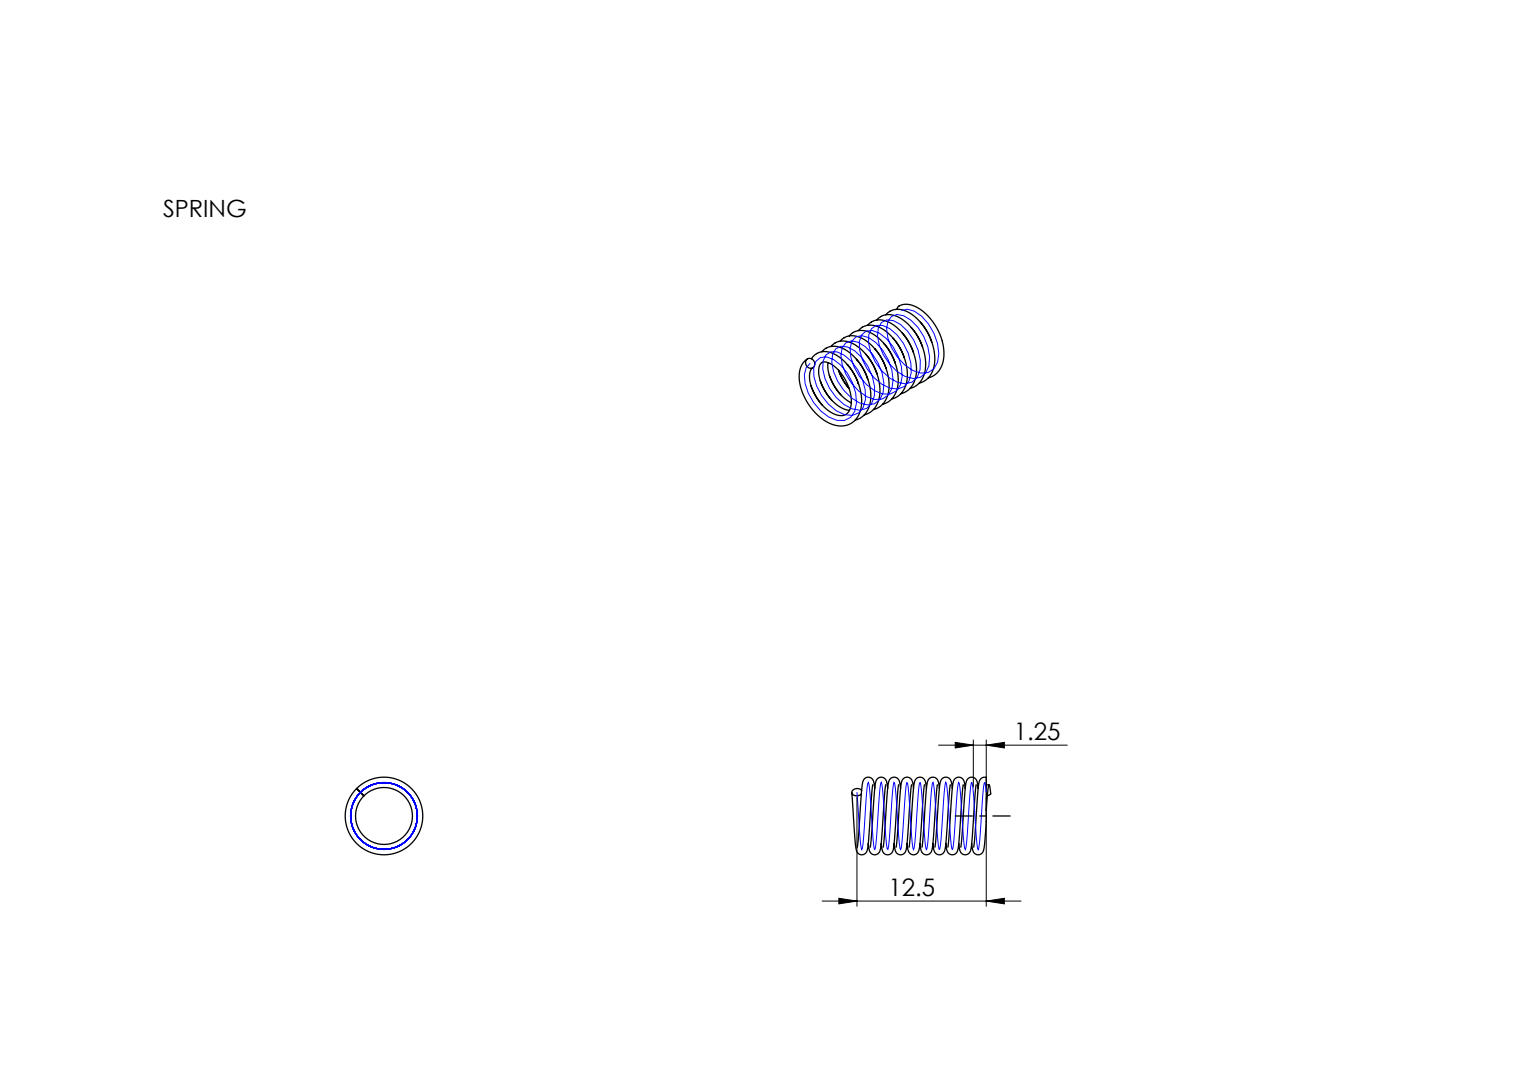
ISO-10303-21;
HEADER;
FILE_DESCRIPTION (('STEP AP214'),
    '1' );
FILE_NAME ('spring.step',
    '2026-10-05T05:16:24',
    ( '' ),
    ( '' ),
    'SwSTEP 2.0',
    'SolidWorks 2026',
    '' );
FILE_SCHEMA (( 'AUTOMOTIVE_DESIGN' ));
ENDSEC;

DATA;
#9=MANIFOLD_SOLID_BREP ( 'Cavity1', #19917 ) ;
#49=CARTESIAN_POINT ( 'NONE',  ( 1.553300858899129944, -11.24999999999998934, 14.70312500000000355 ) ) ;
#65=CARTESIAN_POINT ( 'NONE',  ( 1.200186371490529202, -4.775308065498752974, 18.23624329374151642 ) ) ;
#121=CARTESIAN_POINT ( 'NONE',  ( 2.651650429449539104, -4.848349570550432475, 24.31250000000000000 ) ) ;
#168=CARTESIAN_POINT ( 'NONE',  ( -2.749999999999998224, -7.500000000000015987, 20.09375000000000000 ) ) ;
#179=CARTESIAN_POINT ( 'NONE',  ( 2.750000000000001776, -7.499999999999984013, 18.21875000000000000 ) ) ;
#188=CARTESIAN_POINT ( 'NONE',  ( -2.651650429449565305, -4.848349570550461785, 26.50000000000000355 ) ) ;
#239=CARTESIAN_POINT ( 'NONE',  ( -2.651650429449535551, -10.15165042944956753, 18.68750000000000000 ) ) ;
#270=CARTESIAN_POINT ( 'NONE',  ( -1.987747218494660295, -5.598659921968651254, 17.49813170625848713 ) ) ;
#281=CARTESIAN_POINT ( 'NONE',  ( 1.200186371490561621, -10.22469193450123193, 19.45125670625849068 ) ) ;
#289=CARTESIAN_POINT ( 'NONE',  ( 1.492201783934598236, -11.27530806549875031, 21.20499329374151998 ) ) ;
#294=CARTESIAN_POINT ( 'NONE',  ( 2.608446859217924629, -10.19485399968118422, 24.87686829374151642 ) ) ;
#339=CARTESIAN_POINT ( 'NONE',  ( 1.653273178848927064E-15, -7.500000000000000000, 0.000000000000000000 ) ) ;
#384=CARTESIAN_POINT ( 'NONE',  ( -1.614399933863656544, -3.775308065498769405, 16.32625670625849068 ) ) ;
#392=CARTESIAN_POINT ( 'NONE',  ( -2.608446859217889546, -10.19485399968121264, 18.43563170625848713 ) ) ;
#407=CARTESIAN_POINT ( 'NONE',  ( -2.724691934501246582, -6.299813628509474128, 20.42374329374152353 ) ) ;
#454=CIRCLE ( 'NONE', #72316, 0.4999999999999994449 ) ;
#493=CARTESIAN_POINT ( 'NONE',  ( 1.553300858899087311, -3.749999999999992006, 14.23437500000000355 ) ) ;
#511=CARTESIAN_POINT ( 'NONE',  ( 1.901340078031373171, -9.487747218494639867, 23.62686829374151287 ) ) ;
#518=PRESENTATION_STYLE_ASSIGNMENT (( #82052 ) ) ;
#612=LINE ( 'NONE', #14123, #34562 ) ;
#615=CARTESIAN_POINT ( 'NONE',  ( 1.139087296526029469, -10.24999999999999467, 19.70312500000000355 ) ) ;
#678=CARTESIAN_POINT ( 'NONE',  ( -3.749999999999997335, -7.500000000000021316, 22.59375000000000355 ) ) ;
#710=CARTESIAN_POINT ( 'NONE',  ( -1.901340078031346525, -9.487747218494661183, 19.68563170625849068 ) ) ;
#722=CARTESIAN_POINT ( 'NONE',  ( 1.987747218494664292, -9.401340078031346081, 19.37313170625848713 ) ) ;
#729=CARTESIAN_POINT ( 'NONE',  ( -0.06109907496450878162, -11.25000000000000000, 23.78311829374151998 ) ) ;
#735=CARTESIAN_POINT ( 'NONE',  ( 2.694853999681185108, -4.891553140782077591, 23.31436829374150932 ) ) ;
#817=CARTESIAN_POINT ( 'NONE',  ( -3.749999999999996447, -7.561099074964554134, 17.34188170625849068 ) ) ;
#828=CARTESIAN_POINT ( 'NONE',  ( 0.06109907496455496689, -11.24999999999999822, 15.77938170625848890 ) ) ;
#843=CARTESIAN_POINT ( 'NONE',  ( -2.749999999999999112, -7.438900925035484057, 22.84561829374151642 ) ) ;
#933=CARTESIAN_POINT ( 'NONE',  ( -2.651650429449565305, -4.848349570550461785, 14.00000000000000000 ) ) ;
#939=ORIENTED_EDGE ( 'NONE', *, *, #22476, .F. ) ;
#948=CARTESIAN_POINT ( 'NONE',  ( 1.492201783934598236, -11.27530806549875031, 14.95499329374151642 ) ) ;
#956=CARTESIAN_POINT ( 'NONE',  ( 1.799775606325937360E-14, -10.25000000000000000, 14.78125000000000178 ) ) ;
#1056=CARTESIAN_POINT ( 'NONE',  ( 2.749999999999995115, -6.360912703473971419, 21.89062500000000355 ) ) ;
#1072=CARTESIAN_POINT ( 'NONE',  ( 3.749999999999992006, -5.946699141100872943, 24.39062500000000000 ) ) ;
#1084=ORIENTED_EDGE ( 'NONE', *, *, #14407, .T. ) ;
#1153=CARTESIAN_POINT ( 'NONE',  ( -0.06109907496454585613, -4.750000000000000000, 23.90438170625849068 ) ) ;
#1163=CARTESIAN_POINT ( 'NONE',  ( -1.077988221561460236, -10.27530806549876452, 19.60750670625849068 ) ) ;
#1170=CARTESIAN_POINT ( 'NONE',  ( -2.694853999681181556, -10.10844685921792241, 22.68936829374151287 ) ) ;
#1174=CARTESIAN_POINT ( 'NONE',  ( 3.724691934501251023, -9.114399933863618131, 23.54874329374151642 ) ) ;
#1253=CARTESIAN_POINT ( 'NONE',  ( -1.929879867024197893E-14, -3.750000000000000000, 25.40625000000000000 ) ) ;
#1262=CARTESIAN_POINT ( 'NONE',  ( 3.775308065498768517, -8.992201783934554271, 15.54500670625849246 ) ) ;
#1279=CARTESIAN_POINT ( 'NONE',  ( 2.724691934501250135, -8.700186371490531201, 22.29874329374151642 ) ) ;
#1388=CARTESIAN_POINT ( 'NONE',  ( 1.200186371490529202, -4.775308065498752974, 23.23624329374151642 ) ) ;
#1504=CARTESIAN_POINT ( 'NONE',  ( -2.749999999999991562, -8.639087296526025028, 26.26562500000000000 ) ) ;
#1601=CARTESIAN_POINT ( 'NONE',  ( 2.775308065498768517, -8.577988221561467341, 20.54500670625849068 ) ) ;
#1612=CARTESIAN_POINT ( 'NONE',  ( -0.06109907496454585613, -4.750000000000000000, 25.15438170625849068 ) ) ;
#1621=CARTESIAN_POINT ( 'NONE',  ( -1.553300858899125059, -3.750000000000009326, 15.32812500000000355 ) ) ;
#1630=CARTESIAN_POINT ( 'NONE',  ( -2.651650429449535551, -10.15165042944956753, 17.43750000000000000 ) ) ;
#1705=CARTESIAN_POINT ( 'NONE',  ( 0.06109907496455496689, -11.24999999999999822, 22.02938170625849068 ) ) ;
#1714=CARTESIAN_POINT ( 'NONE',  ( 1.614399933863660985, -11.22469193450123193, 20.70125670625849423 ) ) ;
#1729=CARTESIAN_POINT ( 'NONE',  ( 1.200186371490529202, -4.775308065498752974, 21.98624329374151642 ) ) ;
#1738=ADVANCED_FACE ( 'NONE', ( #45379 ), #86854, .F. ) ;
#1805=CARTESIAN_POINT ( 'NONE',  ( -3.749999999999997335, -7.500000000000021316, 15.09375000000000000 ) ) ;
#1815=CARTESIAN_POINT ( 'NONE',  ( 2.651650429449569302, -10.15165042944953733, 14.62500000000000000 ) ) ;
#1830=CARTESIAN_POINT ( 'NONE',  ( -1.492201783934593573, -3.724691934501250135, 13.07999329374151642 ) ) ;
#1834=CARTESIAN_POINT ( 'NONE',  ( 2.749999999999995115, -6.360912703473971419, 18.14062500000000711 ) ) ;
#1842=CARTESIAN_POINT ( 'NONE',  ( 2.749999999999995115, -6.360912703473971419, 14.39062500000000000 ) ) ;
#1941=CARTESIAN_POINT ( 'NONE',  ( -2.749999999999998224, -7.500000000000015987, 23.84375000000000000 ) ) ;
#2009=CARTESIAN_POINT ( 'NONE',  ( -1.553300858899125059, -3.750000000000009326, 25.32812500000000355 ) ) ;
#2036=CARTESIAN_POINT ( 'NONE',  ( -1.200186371490556958, -4.775308065498765409, 21.32625670625849423 ) ) ;
#2039=CARTESIAN_POINT ( 'NONE',  ( 3.155571303690441365, -7.975156536449540035, 14.00000000000001066 ) ) ;
#2049=CARTESIAN_POINT ( 'NONE',  ( -1.077988221561460236, -10.27530806549876452, 22.10750670625849068 ) ) ;
#2058=CARTESIAN_POINT ( 'NONE',  ( 1.553300858899087311, -3.749999999999992006, 15.48437500000000178 ) ) ;
#2063=CARTESIAN_POINT ( 'NONE',  ( -3.749999999999997335, -7.500000000000021316, 15.09375000000000000 ) ) ;
#2098=CARTESIAN_POINT ( 'NONE',  ( -1.553300858899081538, -11.25000000000000711, 19.85937500000000355 ) ) ;
#2139=CARTESIAN_POINT ( 'NONE',  ( 3.749999999999999556, -7.438900925035446754, 19.21688170625848358 ) ) ;
#2151=CARTESIAN_POINT ( 'NONE',  ( -2.608446859217889546, -10.19485399968121264, 23.43563170625848713 ) ) ;
#2163=CARTESIAN_POINT ( 'NONE',  ( 1.492201783934598236, -11.27530806549875031, 13.70499329374151287 ) ) ;
#2236=CARTESIAN_POINT ( 'NONE',  ( 2.320192649118979489E-14, -11.25000000000000000, 16.03125000000000000 ) ) ;
#2245=CARTESIAN_POINT ( 'NONE',  ( -2.651650429449565305, -4.848349570550461785, 16.50000000000000000 ) ) ;
#2259=CARTESIAN_POINT ( 'NONE',  ( -0.06109907496450878162, -11.25000000000000000, 15.03311829374151287 ) ) ;
#2263=CARTESIAN_POINT ( 'NONE',  ( -2.749999999999991562, -8.639087296526025028, 23.76562499999999645 ) ) ;
#2267=CARTESIAN_POINT ( 'NONE',  ( -1.139087296525992388, -10.25000000000000711, 16.10937500000000355 ) ) ;
#2366=CARTESIAN_POINT ( 'NONE',  ( -2.749999999999998224, -7.500000000000015987, 25.09374999999999645 ) ) ;
#2438=CARTESIAN_POINT ( 'NONE',  ( -3.750000000000007550, -5.946699141100917352, 25.17187500000000000 ) ) ;
#2469=CARTESIAN_POINT ( 'NONE',  ( 2.750000000000001332, -7.438900925035452083, 24.21688170625849068 ) ) ;
#2481=CARTESIAN_POINT ( 'NONE',  ( 1.901340078031349856, -5.512252781505337929, 22.81063170625848713 ) ) ;
#2490=CARTESIAN_POINT ( 'NONE',  ( 2.320192649118979489E-14, -11.25000000000000000, 17.28125000000000000 ) ) ;
#2495=CARTESIAN_POINT ( 'NONE',  ( 1.553300858899129944, -11.24999999999998934, 15.95312500000000000 ) ) ;
#2531=CARTESIAN_POINT ( 'NONE',  ( -3.749999999999988454, -9.053300858899127945, 20.01562500000000355 ) ) ;
#2572=CARTESIAN_POINT ( 'NONE',  ( -2.694853999681210865, -4.891553140782108677, 22.49813170625848713 ) ) ;
#2582=CARTESIAN_POINT ( 'NONE',  ( 1.492201783934554493, -3.724691934501233703, 22.73250670625849068 ) ) ;
#2598=CARTESIAN_POINT ( 'NONE',  ( -2.694853999681181556, -10.10844685921792241, 15.18936829374151465 ) ) ;
#2674=CARTESIAN_POINT ( 'NONE',  ( 2.651650429449569302, -10.15165042944953733, 15.87500000000000000 ) ) ;
#2686=CARTESIAN_POINT ( 'NONE',  ( 2.651650429449539104, -4.848349570550432475, 16.81250000000000000 ) ) ;
#2699=CARTESIAN_POINT ( 'NONE',  ( 3.775308065498752086, -6.007798216065404873, 19.64249329374151642 ) ) ;
#2703=CARTESIAN_POINT ( 'NONE',  ( 1.799775606325937360E-14, -10.25000000000000000, 24.78125000000000000 ) ) ;
#2806=CARTESIAN_POINT ( 'NONE',  ( -1.901340078031369618, -5.512252781505359245, 13.00186829374151465 ) ) ;
#2874=CARTESIAN_POINT ( 'NONE',  ( -1.553300858899081760, -11.25000000000000888, 23.60937500000000711 ) ) ;
#2909=CARTESIAN_POINT ( 'NONE',  ( 2.775308065498768517, -8.577988221561467341, 21.79500670625849068 ) ) ;
#2922=CARTESIAN_POINT ( 'NONE',  ( -2.724691934501232371, -8.700186371490559623, 23.51375670625848713 ) ) ;
#2933=CARTESIAN_POINT ( 'NONE',  ( -1.929879867024197893E-14, -3.750000000000000000, 16.65625000000000000 ) ) ;
#2939=CARTESIAN_POINT ( 'NONE',  ( 1.553300858899129944, -11.24999999999998934, 17.20312500000000000 ) ) ;
#2978=CARTESIAN_POINT ( 'NONE',  ( -1.553300858899081538, -11.25000000000000711, 23.60937500000000711 ) ) ;
#3018=CARTESIAN_POINT ( 'NONE',  ( -3.724691934501229262, -9.114399933863657211, 18.51375670625849068 ) ) ;
#3026=CARTESIAN_POINT ( 'NONE',  ( -3.749999999999996447, -7.561099074964554134, 22.34188170625849068 ) ) ;
#3042=CARTESIAN_POINT ( 'NONE',  ( 1.987747218494642309, -5.598659921968629050, 24.56436829374151287 ) ) ;
#3124=CARTESIAN_POINT ( 'NONE',  ( -3.749999999999997335, -7.500000000000021316, 18.84375000000000000 ) ) ;
#3133=CARTESIAN_POINT ( 'NONE',  ( 3.749999999999992006, -5.946699141100872943, 18.14062500000000711 ) ) ;
#3148=CARTESIAN_POINT ( 'NONE',  ( 2.608446859217924629, -10.19485399968118422, 16.12686829374151287 ) ) ;
#3153=CARTESIAN_POINT ( 'NONE',  ( 1.139087296525997273, -4.749999999999992895, 22.98437500000000000 ) ) ;
#3158=CARTESIAN_POINT ( 'NONE',  ( -1.944543648263014957, -5.555456351737005249, 19.00000000000000000 ) ) ;
#3258=CARTESIAN_POINT ( 'NONE',  ( -2.749999999999999112, -7.438900925035484057, 15.34561829374151465 ) ) ;
#3365=CARTESIAN_POINT ( 'NONE',  ( 2.750000000000008438, -8.639087296525996607, 14.54687500000000178 ) ) ;
#3375=CARTESIAN_POINT ( 'NONE',  ( 2.750000000000001332, -7.438900925035452083, 24.21688170625849068 ) ) ;
#3385=CARTESIAN_POINT ( 'NONE',  ( 1.553300858899129944, -11.24999999999998934, 14.70312500000000355 ) ) ;
#3389=CARTESIAN_POINT ( 'NONE',  ( -3.750000000000008438, -5.946699141100917352, 15.17187500000000000 ) ) ;
#3427=CARTESIAN_POINT ( 'NONE',  ( 2.651650429449539104, -4.848349570550432475, 20.56250000000000000 ) ) ;
#3433=CARTESIAN_POINT ( 'NONE',  ( 3.749999999999992006, -5.946699141100872943, 15.64062500000000178 ) ) ;
#3465=CARTESIAN_POINT ( 'NONE',  ( -2.608446859217889546, -10.19485399968121264, 20.93563170625849068 ) ) ;
#3474=CARTESIAN_POINT ( 'NONE',  ( 0.06109907496455496689, -11.24999999999999822, 22.02938170625849068 ) ) ;
#3487=CARTESIAN_POINT ( 'NONE',  ( 2.608446859217924629, -10.19485399968118422, 16.12686829374151287 ) ) ;
#3569=CARTESIAN_POINT ( 'NONE',  ( 3.749999999999992006, -5.946699141100872943, 14.39062500000000178 ) ) ;
#3579=CARTESIAN_POINT ( 'NONE',  ( 3.750000000000009770, -9.053300858899081760, 17.04687500000000000 ) ) ;
#3594=CARTESIAN_POINT ( 'NONE',  ( 0.06109907496451268821, -3.749999999999999556, 16.90811829374151287 ) ) ;
#3600=CARTESIAN_POINT ( 'NONE',  ( 1.799775606325937360E-14, -10.25000000000000000, 26.03125000000000000 ) ) ;
#3606=CARTESIAN_POINT ( 'NONE',  ( 1.944543648262996083, -5.555456351736983045, 19.31250000000000000 ) ) ;
#3697=CARTESIAN_POINT ( 'NONE',  ( -2.749999999999999112, -7.438900925035484057, 14.09561829374151642 ) ) ;
#3812=CARTESIAN_POINT ( 'NONE',  ( 1.139087296525997273, -4.749999999999992895, 15.48437500000000178 ) ) ;
#3822=CARTESIAN_POINT ( 'NONE',  ( 1.944543648263018731, -9.444543648262994751, 17.12500000000000000 ) ) ;
#3831=CARTESIAN_POINT ( 'NONE',  ( -1.553300858899081538, -11.25000000000000711, 19.85937500000000355 ) ) ;
#3867=CARTESIAN_POINT ( 'NONE',  ( -3.750000000000008438, -5.946699141100917352, 22.67187500000000355 ) ) ;
#3875=CARTESIAN_POINT ( 'NONE',  ( 1.553300858899086867, -3.749999999999992006, 16.73437500000000000 ) ) ;
#3889=CARTESIAN_POINT ( 'NONE',  ( 1.269044939587668397, -4.511073634464840332, 13.80223852175840626 ) ) ;
#3905=CARTESIAN_POINT ( 'NONE',  ( -2.608446859217889546, -10.19485399968121264, 23.43563170625848713 ) ) ;
#3915=CARTESIAN_POINT ( 'NONE',  ( -2.694853999681210865, -4.891553140782108677, 23.74813170625849068 ) ) ;
#3929=CARTESIAN_POINT ( 'NONE',  ( -2.749999999999999112, -7.438900925035484057, 25.34561829374151642 ) ) ;
#4008=CARTESIAN_POINT ( 'NONE',  ( 2.651650429449569302, -10.15165042944953733, 23.37500000000000000 ) ) ;
#4019=CARTESIAN_POINT ( 'NONE',  ( -3.749999999999997335, -7.500000000000021316, 17.59375000000000000 ) ) ;
#4037=CARTESIAN_POINT ( 'NONE',  ( 1.944543648262996083, -5.555456351736983045, 25.56250000000000355 ) ) ;
#4043=CARTESIAN_POINT ( 'NONE',  ( -2.749999999999998224, -7.500000000000015987, 18.84375000000000000 ) ) ;
#4141=CARTESIAN_POINT ( 'NONE',  ( -2.724691934501246582, -6.299813628509474128, 14.17374329374151287 ) ) ;
#4261=CARTESIAN_POINT ( 'NONE',  ( 2.749999999999995115, -6.360912703473971419, 15.64062500000000178 ) ) ;
#4269=CARTESIAN_POINT ( 'NONE',  ( 1.139087296526029469, -10.24999999999999467, 17.20312500000000000 ) ) ;
#4277=CARTESIAN_POINT ( 'NONE',  ( -3.749999999999988454, -9.053300858899127945, 21.26562500000000000 ) ) ;
#4328=CARTESIAN_POINT ( 'NONE',  ( -2.651650429449565305, -4.848349570550461785, 16.50000000000000000 ) ) ;
#4364=CARTESIAN_POINT ( 'NONE',  ( 3.775308065498768517, -8.992201783934554271, 23.04500670625849068 ) ) ;
#4374=CARTESIAN_POINT ( 'NONE',  ( -0.06109907496455085213, -3.750000000000000888, 23.90438170625849068 ) ) ;
#4387=CARTESIAN_POINT ( 'NONE',  ( 2.694853999681185108, -4.891553140782077591, 19.56436829374151287 ) ) ;
#4469=CARTESIAN_POINT ( 'NONE',  ( -3.749999999999997335, -7.500000000000021316, 20.09375000000000000 ) ) ;
#4482=CARTESIAN_POINT ( 'NONE',  ( 1.553300858899129944, -11.24999999999998934, 23.45312500000000000 ) ) ;
#4499=CARTESIAN_POINT ( 'NONE',  ( -2.775308065498752086, -8.577988221561495763, 17.76749329374151287 ) ) ;
#4504=CARTESIAN_POINT ( 'NONE',  ( 1.944543648263018731, -9.444543648262994751, 18.37500000000000355 ) ) ;
#4599=CARTESIAN_POINT ( 'NONE',  ( -2.775308065498752086, -8.577988221561495763, 17.76749329374151287 ) ) ;
#4715=CARTESIAN_POINT ( 'NONE',  ( -1.139087296526025916, -4.750000000000006217, 14.07812500000000178 ) ) ;
#4725=CARTESIAN_POINT ( 'NONE',  ( 1.987747218494664292, -9.401340078031346081, 26.87313170625849423 ) ) ;
#4733=CARTESIAN_POINT ( 'NONE',  ( -1.929879867024197893E-14, -3.750000000000000000, 21.65625000000000355 ) ) ;
#4783=CARTESIAN_POINT ( 'NONE',  ( -3.749999999999997335, -7.500000000000021316, 16.34375000000000000 ) ) ;
#4816=CARTESIAN_POINT ( 'NONE',  ( 2.608446859217893099, -4.805146000318787358, 26.56063170625849068 ) ) ;
#4826=CARTESIAN_POINT ( 'NONE',  ( -1.614399933863656544, -3.775308065498769405, 26.32625670625849068 ) ) ;
#4839=CARTESIAN_POINT ( 'NONE',  ( -3.724691934501248802, -5.885600066136383646, 17.92374329374151287 ) ) ;
#4926=CARTESIAN_POINT ( 'NONE',  ( 2.651650429449569302, -10.15165042944953733, 19.62500000000000000 ) ) ;
#4935=CARTESIAN_POINT ( 'NONE',  ( 2.320192649118979489E-14, -11.25000000000000000, 23.53125000000000000 ) ) ;
#4943=CARTESIAN_POINT ( 'NONE',  ( 2.952004793765244717, -6.965521097154411478, 14.00000000000000178 ) ) ;
#4951=CARTESIAN_POINT ( 'NONE',  ( 1.987747218494642309, -5.598659921968629050, 15.81436829374151465 ) ) ;
#4956=CARTESIAN_POINT ( 'NONE',  ( 1.944543648262996083, -5.555456351736983045, 16.81250000000000000 ) ) ;
#5043=CARTESIAN_POINT ( 'NONE',  ( 1.200186371490529202, -4.775308065498752974, 15.73624329374151998 ) ) ;
#5153=CARTESIAN_POINT ( 'NONE',  ( 2.750000000000001332, -7.438900925035452083, 25.46688170625849423 ) ) ;
#5162=CARTESIAN_POINT ( 'NONE',  ( 1.077988221561464899, -4.724691934501233703, 26.48250670625848713 ) ) ;
#5171=CARTESIAN_POINT ( 'NONE',  ( 3.750000000000009770, -9.053300858899081760, 22.04687500000000000 ) ) ;
#5214=CARTESIAN_POINT ( 'NONE',  ( 3.750000000000000888, -7.499999999999978684, 25.71875000000000000 ) ) ;
#5252=CARTESIAN_POINT ( 'NONE',  ( -1.987747218494660295, -5.598659921968651254, 14.99813170625848713 ) ) ;
#5265=CARTESIAN_POINT ( 'NONE',  ( 1.614399933863660985, -11.22469193450123193, 24.45125670625849423 ) ) ;
#5274=CARTESIAN_POINT ( 'NONE',  ( -1.614399933863613468, -11.22469193450124969, 20.11124329374151642 ) ) ;
#5280=CARTESIAN_POINT ( 'NONE',  ( 3.724691934501251023, -9.114399933863618131, 18.54874329374151642 ) ) ;
#5366=CARTESIAN_POINT ( 'NONE',  ( -1.929879867024197893E-14, -3.750000000000000000, 20.40625000000000000 ) ) ;
#5375=CARTESIAN_POINT ( 'NONE',  ( -3.749999999999988454, -9.053300858899127945, 25.01562500000000000 ) ) ;
#5395=CARTESIAN_POINT ( 'NONE',  ( 1.901340078031373171, -9.487747218494639867, 18.62686829374151642 ) ) ;
#5402=CARTESIAN_POINT ( 'NONE',  ( -1.139087296525992388, -10.25000000000000711, 24.85937500000000711 ) ) ;
#5500=CARTESIAN_POINT ( 'NONE',  ( 1.901340078031373171, -9.487747218494639867, 21.12686829374151287 ) ) ;
#5599=CARTESIAN_POINT ( 'NONE',  ( 2.749999999999995115, -6.360912703473971419, 19.39062500000000711 ) ) ;
#5608=CARTESIAN_POINT ( 'NONE',  ( -1.077988221561460236, -10.27530806549876452, 27.10750670625849423 ) ) ;
#5615=CARTESIAN_POINT ( 'NONE',  ( 2.320192649118979489E-14, -11.25000000000000000, 23.53125000000000000 ) ) ;
#5661=CARTESIAN_POINT ( 'NONE',  ( 3.750000000000009770, -9.053300858899081760, 19.54687500000000000 ) ) ;
#5691=CARTESIAN_POINT ( 'NONE',  ( 0.06109907496455496689, -11.24999999999999822, 23.27938170625849068 ) ) ;
#5707=CARTESIAN_POINT ( 'NONE',  ( -2.608446859217889546, -10.19485399968121264, 25.93563170625849423 ) ) ;
#5715=CARTESIAN_POINT ( 'NONE',  ( 2.608446859217924629, -10.19485399968118422, 17.37686829374151287 ) ) ;
#5721=CARTESIAN_POINT ( 'NONE',  ( 0.06109907496451268821, -3.749999999999999556, 18.15811829374151642 ) ) ;
#5808=CARTESIAN_POINT ( 'NONE',  ( -3.750000000000008438, -5.946699141100917352, 21.42187500000000000 ) ) ;
#5818=CARTESIAN_POINT ( 'NONE',  ( 3.749999999999992006, -5.946699141100872943, 23.14062500000000000 ) ) ;
#5833=CARTESIAN_POINT ( 'NONE',  ( -1.200186371490524317, -10.22469193450124791, 15.11124329374151287 ) ) ;
#5842=CARTESIAN_POINT ( 'NONE',  ( -1.139087296526025250, -4.750000000000006217, 22.82812500000000355 ) ) ;
#5942=CARTESIAN_POINT ( 'NONE',  ( -2.749999999999999112, -7.438900925035484057, 20.34561829374151287 ) ) ;
#6049=CARTESIAN_POINT ( 'NONE',  ( 1.944543648263018731, -9.444543648262994751, 20.87500000000000000 ) ) ;
#6057=CARTESIAN_POINT ( 'NONE',  ( 1.139087296525997273, -4.749999999999992895, 19.23437500000000355 ) ) ;
#6066=CARTESIAN_POINT ( 'NONE',  ( -1.553300858899125059, -3.750000000000009326, 24.07812500000000355 ) ) ;
#6114=CARTESIAN_POINT ( 'NONE',  ( 3.750000000000000888, -7.499999999999978684, 21.96875000000000355 ) ) ;
#6140=CARTESIAN_POINT ( 'NONE',  ( 1.200186371490561621, -10.22469193450123193, 16.95125670625848713 ) ) ;
#6154=CARTESIAN_POINT ( 'NONE',  ( -2.775308065498764964, -6.422011778438537988, 16.17000670625848713 ) ) ;
#6163=CARTESIAN_POINT ( 'NONE',  ( 3.775308065498752086, -6.007798216065404873, 23.39249329374151642 ) ) ;
#6168=CARTESIAN_POINT ( 'NONE',  ( -2.608446859217920633, -4.805146000318815780, 19.25186829374151287 ) ) ;
#6259=CARTESIAN_POINT ( 'NONE',  ( -3.749999999999996447, -7.561099074964554134, 16.09188170625848713 ) ) ;
#6267=CARTESIAN_POINT ( 'NONE',  ( -1.553300858899081538, -11.25000000000000711, 21.10937500000000711 ) ) ;
#6282=CARTESIAN_POINT ( 'NONE',  ( 0.06109907496451789238, -4.749999999999998224, 16.90811829374151287 ) ) ;
#6291=CARTESIAN_POINT ( 'NONE',  ( 1.799775606325937360E-14, -10.25000000000000000, 22.28125000000000355 ) ) ;
#6391=CARTESIAN_POINT ( 'NONE',  ( -0.06109907496451398579, -10.25000000000000178, 22.53311829374151642 ) ) ;
#6395=SURFACE_STYLE_FILL_AREA ( #48245 ) ;
#6490=CARTESIAN_POINT ( 'NONE',  ( -2.749999999999991562, -8.639087296526025028, 18.76562500000000000 ) ) ;
#6498=CARTESIAN_POINT ( 'NONE',  ( -1.409462824231155764E-14, -4.749999999999999112, 17.90625000000000000 ) ) ;
#6507=CARTESIAN_POINT ( 'NONE',  ( 2.651650429449539104, -4.848349570550432475, 24.31250000000000000 ) ) ;
#6556=CARTESIAN_POINT ( 'NONE',  ( -1.553300858899081760, -11.25000000000000888, 22.35937500000000355 ) ) ;
#6586=CARTESIAN_POINT ( 'NONE',  ( 0.06109907496454976272, -10.25000000000000000, 18.27938170625849068 ) ) ;
#6598=CARTESIAN_POINT ( 'NONE',  ( -1.901340078031346525, -9.487747218494661183, 17.18563170625848713 ) ) ;
#6604=CARTESIAN_POINT ( 'NONE',  ( -2.121320343559653487, -5.378679656440369605, 14.00000000000000178 ) ) ;
#6605=CARTESIAN_POINT ( 'NONE',  ( -2.608446859217920633, -4.805146000318815780, 24.25186829374150932 ) ) ;
#6610=CARTESIAN_POINT ( 'NONE',  ( -3.749999999999997780, -7.438900925035489387, 25.34561829374151642 ) ) ;
#6688=CARTESIAN_POINT ( 'NONE',  ( -1.553300858899081538, -11.25000000000000711, 24.85937500000001421 ) ) ;
#6696=CARTESIAN_POINT ( 'NONE',  ( 3.749999999999999556, -7.438900925035446754, 17.96688170625848713 ) ) ;
#6711=CARTESIAN_POINT ( 'NONE',  ( -2.724691934501246582, -6.299813628509474128, 21.67374329374151287 ) ) ;
#6719=CARTESIAN_POINT ( 'NONE',  ( 1.944543648262996083, -5.555456351736983045, 25.56250000000000355 ) ) ;
#6813=CARTESIAN_POINT ( 'NONE',  ( -2.749999999999999112, -7.438900925035484057, 22.84561829374151642 ) ) ;
#6871=CARTESIAN_POINT ( 'NONE',  ( 3.750000000000000888, -7.499999999999978684, 24.46875000000000000 ) ) ;
#6920=CARTESIAN_POINT ( 'NONE',  ( -2.749999999999991562, -8.639087296526025028, 17.51562500000000000 ) ) ;
#6931=CARTESIAN_POINT ( 'NONE',  ( -2.749999999999991562, -8.639087296526025028, 22.51562500000000000 ) ) ;
#6994=CARTESIAN_POINT ( 'NONE',  ( 1.553300858899129722, -11.24999999999999112, 18.45312499999999645 ) ) ;
#7021=CARTESIAN_POINT ( 'NONE',  ( -2.724691934501232371, -8.700186371490559623, 17.26375670625849068 ) ) ;
#7033=CARTESIAN_POINT ( 'NONE',  ( -1.200186371490556958, -4.775308065498765409, 18.82625670625848713 ) ) ;
#7042=CARTESIAN_POINT ( 'NONE',  ( 3.724691934501251023, -9.114399933863618131, 24.79874329374151998 ) ) ;
#7050=CARTESIAN_POINT ( 'NONE',  ( 3.775308065498752086, -6.007798216065404873, 23.39249329374151642 ) ) ;
#7137=CARTESIAN_POINT ( 'NONE',  ( 2.694853999681214862, -10.10844685921789043, 15.62313170625848890 ) ) ;
#7145=CARTESIAN_POINT ( 'NONE',  ( 3.775308065498768517, -8.992201783934554271, 16.79500670625849068 ) ) ;
#7162=CARTESIAN_POINT ( 'NONE',  ( -1.987747218494638313, -9.401340078031370950, 23.93936829374151642 ) ) ;
#7169=CARTESIAN_POINT ( 'NONE',  ( -2.749999999999991562, -8.639087296526026805, 22.51562500000000000 ) ) ;
#7252=CARTESIAN_POINT ( 'NONE',  ( 3.750000000000000888, -7.499999999999978684, 14.46875000000000000 ) ) ;
#7268=CARTESIAN_POINT ( 'NONE',  ( -1.901340078031369618, -5.512252781505359245, 19.25186829374151287 ) ) ;
#7326=CARTESIAN_POINT ( 'NONE',  ( 2.320192649118979489E-14, -11.25000000000000000, 24.78125000000000000 ) ) ;
#7378=CARTESIAN_POINT ( 'NONE',  ( -1.944543648262992530, -9.444543648263016067, 18.68750000000000000 ) ) ;
#7395=CARTESIAN_POINT ( 'NONE',  ( -1.553300858899125059, -3.750000000000009326, 25.32812500000000711 ) ) ;
#7445=CARTESIAN_POINT ( 'NONE',  ( 2.320192649118979489E-14, -11.25000000000000000, 21.03125000000000000 ) ) ;
#7477=CARTESIAN_POINT ( 'NONE',  ( -1.200186371490556958, -4.775308065498765409, 17.57625670625849068 ) ) ;
#7489=CARTESIAN_POINT ( 'NONE',  ( 1.077988221561464899, -4.724691934501233703, 16.48250670625849423 ) ) ;
#7497=CARTESIAN_POINT ( 'NONE',  ( -1.614399933863613468, -11.22469193450124969, 21.36124329374151642 ) ) ;
#7502=CARTESIAN_POINT ( 'NONE',  ( -2.694853999681181556, -10.10844685921792241, 22.68936829374151287 ) ) ;
#7568=AXIS2_PLACEMENT_3D ( 'NONE', #37517, #16371, #65873 ) ;
#7582=CARTESIAN_POINT ( 'NONE',  ( -3.724691934501229262, -9.114399933863657211, 17.26375670625849068 ) ) ;
#7591=CARTESIAN_POINT ( 'NONE',  ( 1.492201783934554493, -3.724691934501233703, 15.23250670625848713 ) ) ;
#7607=CARTESIAN_POINT ( 'NONE',  ( 1.987747218494642309, -5.598659921968629050, 20.81436829374151287 ) ) ;
#7614=CARTESIAN_POINT ( 'NONE',  ( -1.944543648263015179, -5.555456351737005249, 26.50000000000000355 ) ) ;
#7701=CARTESIAN_POINT ( 'NONE',  ( -2.651650429449565305, -4.848349570550461785, 15.25000000000000000 ) ) ;
#7718=CARTESIAN_POINT ( 'NONE',  ( 2.608446859217924629, -10.19485399968118422, 14.87686829374151465 ) ) ;
#7725=CARTESIAN_POINT ( 'NONE',  ( -1.139087296525992388, -10.25000000000000711, 14.85937500000000355 ) ) ;
#7816=CARTESIAN_POINT ( 'NONE',  ( 1.944543648263018731, -9.444543648262994751, 23.37500000000000000 ) ) ;
#7832=CARTESIAN_POINT ( 'NONE',  ( 2.651650429449569302, -10.15165042944953733, 25.87500000000000355 ) ) ;
#7915=CARTESIAN_POINT ( 'NONE',  ( -2.749999999999997780, -7.561099074964547917, 18.59188170625849068 ) ) ;
#7927=CARTESIAN_POINT ( 'NONE',  ( -1.901340078031346525, -9.487747218494661183, 18.43563170625848713 ) ) ;
#7934=CARTESIAN_POINT ( 'NONE',  ( 2.608446859217924629, -10.19485399968118422, 23.62686829374151287 ) ) ;
#7940=CARTESIAN_POINT ( 'NONE',  ( -3.749999999999997780, -7.438900925035489387, 21.59561829374151287 ) ) ;
#8024=CARTESIAN_POINT ( 'NONE',  ( 2.320192649118979489E-14, -11.25000000000000000, 26.03125000000000000 ) ) ;
#8033=CARTESIAN_POINT ( 'NONE',  ( -1.929879867024197893E-14, -3.750000000000000000, 25.40625000000000000 ) ) ;
#8050=CARTESIAN_POINT ( 'NONE',  ( 0.06109907496451789238, -4.749999999999998224, 20.65811829374151287 ) ) ;
#8155=CARTESIAN_POINT ( 'NONE',  ( -1.614399933863613468, -11.22469193450124969, 13.86124329374151820 ) ) ;
#8265=CARTESIAN_POINT ( 'NONE',  ( -1.139087296526025916, -4.750000000000006217, 24.07812500000000355 ) ) ;
#8362=CARTESIAN_POINT ( 'NONE',  ( 2.724691934501235036, -6.299813628509441266, 24.13875670625849068 ) ) ;
#8364=CARTESIAN_POINT ( 'NONE',  ( -1.790671178605550695, -4.201618623452029411, 14.00000000000000711 ) ) ;
#8373=CARTESIAN_POINT ( 'NONE',  ( -1.200186371490556958, -4.775308065498765409, 25.07625670625849423 ) ) ;
#8381=CARTESIAN_POINT ( 'NONE',  ( 2.320192649118979489E-14, -11.25000000000000000, 14.78125000000000178 ) ) ;
#8386=CARTESIAN_POINT ( 'NONE',  ( 3.775308065498752086, -6.007798216065404873, 22.14249329374151998 ) ) ;
#8470=CARTESIAN_POINT ( 'NONE',  ( 3.775308065498768517, -8.992201783934554271, 21.79500670625849068 ) ) ;
#8479=CARTESIAN_POINT ( 'NONE',  ( -3.724691934501229262, -9.114399933863657211, 17.26375670625849068 ) ) ;
#8494=CARTESIAN_POINT ( 'NONE',  ( -1.200186371490524317, -10.22469193450124791, 22.61124329374151287 ) ) ;
#8599=CARTESIAN_POINT ( 'NONE',  ( -1.077988221561493543, -4.724691934501247914, 23.07999329374151998 ) ) ;
#8605=CARTESIAN_POINT ( 'NONE',  ( -2.750000000000007105, -6.360912703474006946, 21.42187500000000000 ) ) ;
#8708=CARTESIAN_POINT ( 'NONE',  ( 1.799775606325937360E-14, -10.25000000000000000, 24.78125000000000000 ) ) ;
#8775=CARTESIAN_POINT ( 'NONE',  ( -2.651650429449565305, -4.848349570550461785, 25.25000000000000000 ) ) ;
#8807=CARTESIAN_POINT ( 'NONE',  ( 1.200186371490561621, -10.22469193450123193, 20.70125670625849423 ) ) ;
#8809=CARTESIAN_POINT ( 'NONE',  ( 3.432150206517289082, -7.475741165495100482, 14.00000000000201794 ) ) ;
#8818=CARTESIAN_POINT ( 'NONE',  ( -0.06109907496454585613, -4.750000000000000000, 21.40438170625849068 ) ) ;
#8828=CARTESIAN_POINT ( 'NONE',  ( -2.651650429449565305, -4.848349570550461785, 16.50000000000000000 ) ) ;
#8834=CARTESIAN_POINT ( 'NONE',  ( -2.651650429449535551, -10.15165042944956753, 18.68750000000000000 ) ) ;
#8871=CARTESIAN_POINT ( 'NONE',  ( -2.651650429449565305, -4.848349570550461785, 20.25000000000000000 ) ) ;
#8912=CARTESIAN_POINT ( 'NONE',  ( 1.614399933863660985, -11.22469193450123193, 20.70125670625849423 ) ) ;
#8924=CARTESIAN_POINT ( 'NONE',  ( 2.694853999681214862, -10.10844685921789043, 19.37313170625848713 ) ) ;
#8937=CARTESIAN_POINT ( 'NONE',  ( -2.775308065498752086, -8.577988221561495763, 25.26749329374151642 ) ) ;
#9018=CARTESIAN_POINT ( 'NONE',  ( -3.749999999999997335, -7.500000000000021316, 17.59375000000000000 ) ) ;
#9030=CARTESIAN_POINT ( 'NONE',  ( -3.749999999999997335, -7.500000000000021316, 16.34375000000000000 ) ) ;
#9043=CARTESIAN_POINT ( 'NONE',  ( 0.06109907496451268821, -3.749999999999999556, 13.15811829374151642 ) ) ;
#9047=CARTESIAN_POINT ( 'NONE',  ( 1.799775606325937360E-14, -10.25000000000000000, 21.03125000000000000 ) ) ;
#9154=CARTESIAN_POINT ( 'NONE',  ( -1.944543648262992530, -9.444543648263016067, 22.43750000000000000 ) ) ;
#9220=CARTESIAN_POINT ( 'NONE',  ( -2.651650429449565305, -4.848349570550461785, 26.50000000000000355 ) ) ;
#9255=CARTESIAN_POINT ( 'NONE',  ( 2.724691934501235036, -6.299813628509441266, 20.38875670625849068 ) ) ;
#9258=CARTESIAN_POINT ( 'NONE',  ( 3.271582784339720273, -7.991356743646568006, 14.00000000000000533 ) ) ;
#9265=CARTESIAN_POINT ( 'NONE',  ( 1.987747218494664292, -9.401340078031346081, 25.62313170625849068 ) ) ;
#9273=CARTESIAN_POINT ( 'NONE',  ( -3.749999999999988454, -9.053300858899127945, 16.26562500000000000 ) ) ;
#9277=CARTESIAN_POINT ( 'NONE',  ( -1.929879867024197893E-14, -3.750000000000000000, 16.65625000000000000 ) ) ;
#9315=CARTESIAN_POINT ( 'NONE',  ( 3.749999999999992006, -5.946699141100872943, 21.89062500000000355 ) ) ;
#9357=CARTESIAN_POINT ( 'NONE',  ( -2.694853999681210865, -4.891553140782108677, 21.24813170625848713 ) ) ;
#9366=CARTESIAN_POINT ( 'NONE',  ( -3.749999999999996447, -7.561099074964554134, 21.09188170625849068 ) ) ;
#9378=CARTESIAN_POINT ( 'NONE',  ( 3.750000000000001776, -7.561099074964511502, 14.72061829374151465 ) ) ;
#9419=ORIENTED_EDGE ( 'NONE', *, *, #14407, .F. ) ;
#9451=CARTESIAN_POINT ( 'NONE',  ( 2.651650429449569302, -10.15165042944953733, 14.62500000000000000 ) ) ;
#9461=CARTESIAN_POINT ( 'NONE',  ( 2.651650429449539104, -4.848349570550432475, 15.56250000000000000 ) ) ;
#9473=CARTESIAN_POINT ( 'NONE',  ( -1.987747218494638313, -9.401340078031370950, 23.93936829374151642 ) ) ;
#9477=CARTESIAN_POINT ( 'NONE',  ( -2.749999999999998224, -7.500000000000015987, 26.34375000000000000 ) ) ;
#9575=CARTESIAN_POINT ( 'NONE',  ( -1.944543648262992530, -9.444543648263016067, 23.68750000000000000 ) ) ;
#9681=CARTESIAN_POINT ( 'NONE',  ( -2.749999999999997780, -7.561099074964547917, 21.09188170625849068 ) ) ;
#9691=CARTESIAN_POINT ( 'NONE',  ( -2.775308065498764964, -6.422011778438537988, 24.92000670625849068 ) ) ;
#9699=CARTESIAN_POINT ( 'NONE',  ( -1.929879867024197893E-14, -3.750000000000000000, 15.40625000000000000 ) ) ;
#9704=CARTESIAN_POINT ( 'NONE',  ( -2.651650429449535551, -10.15165042944956753, 14.93750000000000000 ) ) ;
#9744=CARTESIAN_POINT ( 'NONE',  ( 2.651650429449569302, -10.15165042944953733, 23.37500000000000000 ) ) ;
#9787=CARTESIAN_POINT ( 'NONE',  ( -1.614399933863656544, -3.775308065498769405, 18.82625670625848713 ) ) ;
#9796=CARTESIAN_POINT ( 'NONE',  ( 3.724691934501232815, -5.885600066136343678, 20.38875670625849068 ) ) ;
#9809=CARTESIAN_POINT ( 'NONE',  ( 3.750000000000001776, -7.561099074964511502, 15.97061829374151287 ) ) ;
#9890=CARTESIAN_POINT ( 'NONE',  ( 1.553300858899087311, -3.749999999999992006, 15.48437500000000178 ) ) ;
#9900=CARTESIAN_POINT ( 'NONE',  ( -3.749999999999997335, -7.500000000000021316, 20.09375000000000000 ) ) ;
#9913=CARTESIAN_POINT ( 'NONE',  ( -0.06109907496450878162, -11.25000000000000000, 20.03311829374151287 ) ) ;
#9919=CARTESIAN_POINT ( 'NONE',  ( -0.06109907496451398579, -10.25000000000000178, 13.78311829374151287 ) ) ;
#9923=CARTESIAN_POINT ( 'NONE',  ( 1.799775606325937360E-14, -10.25000000000000000, 19.78125000000000000 ) ) ;
#10018=CARTESIAN_POINT ( 'NONE',  ( 2.724691934501250135, -8.700186371490531201, 16.04874329374151287 ) ) ;
#10128=CARTESIAN_POINT ( 'NONE',  ( 1.901340078031349856, -5.512252781505337929, 20.31063170625848713 ) ) ;
#10141=CARTESIAN_POINT ( 'NONE',  ( -1.901340078031346525, -9.487747218494661183, 25.93563170625849423 ) ) ;
#10153=CARTESIAN_POINT ( 'NONE',  ( -2.651650429449535551, -10.15165042944956753, 14.93750000000000000 ) ) ;
#10158=CARTESIAN_POINT ( 'NONE',  ( 2.651650429449569302, -10.15165042944953733, 18.37500000000000355 ) ) ;
#10197=CARTESIAN_POINT ( 'NONE',  ( -3.750000000000008438, -5.946699141100917352, 21.42187500000000000 ) ) ;
#10221=CARTESIAN_POINT ( 'NONE',  ( 2.787413173340201222, -6.056457615119054338, 13.93844569653987087 ) ) ;
#10241=CARTESIAN_POINT ( 'NONE',  ( -1.614399933863656544, -3.775308065498769405, 20.07625670625849068 ) ) ;
#10249=CARTESIAN_POINT ( 'NONE',  ( 3.749999999999999556, -7.438900925035446754, 19.21688170625848358 ) ) ;
#10263=CARTESIAN_POINT ( 'NONE',  ( 1.492201783934598236, -11.27530806549875031, 14.95499329374151642 ) ) ;
#10340=CARTESIAN_POINT ( 'NONE',  ( 1.553300858899087311, -3.749999999999992006, 19.23437500000000355 ) ) ;
#10349=CARTESIAN_POINT ( 'NONE',  ( -2.651650429449535551, -10.15165042944956753, 17.43750000000000000 ) ) ;
#10366=CARTESIAN_POINT ( 'NONE',  ( -0.06109907496450878162, -11.25000000000000000, 16.28311829374151287 ) ) ;
#10373=CARTESIAN_POINT ( 'NONE',  ( -2.749999999999998224, -7.500000000000015987, 25.09374999999999645 ) ) ;
#10377=CARTESIAN_POINT ( 'NONE',  ( 1.799775606325937360E-14, -10.25000000000000000, 17.28125000000000000 ) ) ;
#10474=CARTESIAN_POINT ( 'NONE',  ( 1.200186371490529202, -4.775308065498752974, 16.98624329374151287 ) ) ;
#10579=CARTESIAN_POINT ( 'NONE',  ( -1.139087296526025916, -4.750000000000006217, 15.32812500000000355 ) ) ;
#10583=CARTESIAN_POINT ( 'NONE',  ( 3.148534467955792948, -7.948670516411742604, 14.00000000000001066 ) ) ;
#10591=CARTESIAN_POINT ( 'NONE',  ( 2.750000000000001776, -7.499999999999984013, 16.96875000000000000 ) ) ;
#10599=CARTESIAN_POINT ( 'NONE',  ( -3.750000000000008438, -5.946699141100917352, 20.17187500000000000 ) ) ;
#10641=CARTESIAN_POINT ( 'NONE',  ( 1.553300858899087311, -3.749999999999992006, 21.73437500000000000 ) ) ;
#10647=CARTESIAN_POINT ( 'NONE',  ( -1.553300858899125059, -3.750000000000009326, 17.82812500000000000 ) ) ;
#10680=CARTESIAN_POINT ( 'NONE',  ( 3.749999999999999556, -7.438900925035446754, 26.71688170625849068 ) ) ;
#10690=CARTESIAN_POINT ( 'NONE',  ( 3.724691934501232815, -5.885600066136343678, 24.13875670625849068 ) ) ;
#10703=CARTESIAN_POINT ( 'NONE',  ( 2.608446859217924629, -10.19485399968118422, 14.87686829374151465 ) ) ;
#10784=CARTESIAN_POINT ( 'NONE',  ( 1.553300858899087311, -3.749999999999992006, 21.73437500000000000 ) ) ;
#10794=CARTESIAN_POINT ( 'NONE',  ( 1.553300858899129944, -11.24999999999998934, 15.95312500000000000 ) ) ;
#10814=CARTESIAN_POINT ( 'NONE',  ( 1.944543648262996083, -5.555456351736983045, 23.06250000000000000 ) ) ;
#10821=CARTESIAN_POINT ( 'NONE',  ( 2.750000000000008438, -8.639087296525996607, 20.79687500000000000 ) ) ;
#10915=CARTESIAN_POINT ( 'NONE',  ( 2.724691934501250135, -8.700186371490531201, 17.29874329374151642 ) ) ;
#11000=SHAPE_REPRESENTATION ( 'spring', ( #83448 ), #34517 ) ;
#11025=CARTESIAN_POINT ( 'NONE',  ( 1.944543648262996083, -5.555456351736983045, 15.56250000000000000 ) ) ;
#11034=CARTESIAN_POINT ( 'NONE',  ( -1.139087296525992166, -10.25000000000000533, 14.85937500000000355 ) ) ;
#11042=CARTESIAN_POINT ( 'NONE',  ( -3.749999999999997335, -7.500000000000021316, 21.34375000000000000 ) ) ;
#11090=CARTESIAN_POINT ( 'NONE',  ( -3.749999999999988454, -9.053300858899127945, 15.01562500000000178 ) ) ;
#11120=CARTESIAN_POINT ( 'NONE',  ( -2.694853999681210865, -4.891553140782108677, 23.74813170625849068 ) ) ;
#11128=CARTESIAN_POINT ( 'NONE',  ( 2.775308065498768517, -8.577988221561467341, 15.54500670625849246 ) ) ;
#11143=CARTESIAN_POINT ( 'NONE',  ( 1.614399933863618797, -3.775308065498751198, 16.98624329374151287 ) ) ;
#11226=CARTESIAN_POINT ( 'NONE',  ( -2.298097038856290464, -5.201902961143733961, 26.50000000000000355 ) ) ;
#11230=CARTESIAN_POINT ( 'NONE',  ( -1.553300858899125059, -3.750000000000009326, 22.82812500000000355 ) ) ;
#11239=CARTESIAN_POINT ( 'NONE',  ( 3.750000000000000888, -7.499999999999978684, 24.46875000000000000 ) ) ;
#11257=CARTESIAN_POINT ( 'NONE',  ( 1.944543648263018731, -9.444543648262994751, 23.37500000000000000 ) ) ;
#11263=CARTESIAN_POINT ( 'NONE',  ( 2.749999999999995115, -6.360912703473971419, 19.39062500000000355 ) ) ;
#11354=CARTESIAN_POINT ( 'NONE',  ( -1.200186371490524317, -10.22469193450124791, 17.61124329374151642 ) ) ;
#11470=CARTESIAN_POINT ( 'NONE',  ( 2.750000000000001776, -7.499999999999984013, 15.71875000000000000 ) ) ;
#11478=CARTESIAN_POINT ( 'NONE',  ( -2.749999999999991562, -8.639087296526025028, 17.51562500000000000 ) ) ;
#11487=CARTESIAN_POINT ( 'NONE',  ( 2.320192649118979489E-14, -11.25000000000000000, 21.03125000000000000 ) ) ;
#11512=ADVANCED_FACE ( 'NONE', ( #74184 ), #16029, .F. ) ;
#11538=CARTESIAN_POINT ( 'NONE',  ( 3.750000000000009770, -9.053300858899081760, 14.54687500000000000 ) ) ;
#11574=CARTESIAN_POINT ( 'NONE',  ( -3.724691934501229262, -9.114399933863657211, 23.51375670625848713 ) ) ;
#11583=CARTESIAN_POINT ( 'NONE',  ( 1.614399933863660985, -11.22469193450123193, 26.95125670625849068 ) ) ;
#11598=CARTESIAN_POINT ( 'NONE',  ( -3.775308065498748977, -8.992201783934593351, 19.01749329374151287 ) ) ;
#11683=CARTESIAN_POINT ( 'NONE',  ( 3.750000000000000888, -7.499999999999978684, 23.21875000000000000 ) ) ;
#11693=CARTESIAN_POINT ( 'NONE',  ( 2.651650429449569302, -10.15165042944953733, 22.12500000000000000 ) ) ;
#11711=CARTESIAN_POINT ( 'NONE',  ( -2.749999999999999112, -7.438900925035484057, 14.09561829374151642 ) ) ;
#11718=CARTESIAN_POINT ( 'NONE',  ( -1.139087296525992388, -10.25000000000000711, 18.60937500000000355 ) ) ;
#11810=CARTESIAN_POINT ( 'NONE',  ( 2.775308065498755195, -6.422011778438505125, 13.39249329374151642 ) ) ;
#11850=ORIENTED_EDGE ( 'NONE', *, *, #38124, .T. ) ;
#11921=CARTESIAN_POINT ( 'NONE',  ( -1.944543648263014957, -5.555456351737005249, 16.50000000000000000 ) ) ;
#11931=CARTESIAN_POINT ( 'NONE',  ( 2.750000000000001776, -7.499999999999984013, 14.46875000000000000 ) ) ;
#11940=CARTESIAN_POINT ( 'NONE',  ( 1.553300858899087311, -3.749999999999992006, 19.23437500000000355 ) ) ;
#11973=EDGE_CURVE ( 'NONE', #25338, #61929, #82093, .T. ) ;
#11990=CARTESIAN_POINT ( 'NONE',  ( -1.553300858899125059, -3.750000000000009326, 14.07812500000000178 ) ) ;
#12021=CARTESIAN_POINT ( 'NONE',  ( -2.694853999681210865, -4.891553140782108677, 27.49813170625849068 ) ) ;
#12033=CARTESIAN_POINT ( 'NONE',  ( 2.608446859217893099, -4.805146000318787358, 25.31063170625848713 ) ) ;
#12043=CARTESIAN_POINT ( 'NONE',  ( -2.608446859217920633, -4.805146000318815780, 15.50186829374151287 ) ) ;
#12050=CARTESIAN_POINT ( 'NONE',  ( -1.614399933863613468, -11.22469193450124969, 17.61124329374151642 ) ) ;
#12129=CARTESIAN_POINT ( 'NONE',  ( 3.749999999999992006, -5.946699141100872943, 21.89062500000000355 ) ) ;
#12139=CARTESIAN_POINT ( 'NONE',  ( -3.749999999999997335, -7.500000000000021316, 23.84375000000000000 ) ) ;
#12154=CARTESIAN_POINT ( 'NONE',  ( 2.724691934501250135, -8.700186371490531201, 18.54874329374151642 ) ) ;
#12159=CARTESIAN_POINT ( 'NONE',  ( -1.139087296525992388, -10.25000000000000711, 22.35937500000000355 ) ) ;
#12247=CARTESIAN_POINT ( 'NONE',  ( 1.987747218494642309, -5.598659921968629050, 20.81436829374151287 ) ) ;
#12335=CARTESIAN_POINT ( 'NONE',  ( 1.553300858899087311, -3.749999999999992006, 14.23437500000000355 ) ) ;
#12359=CARTESIAN_POINT ( 'NONE',  ( 1.139087296525997273, -4.749999999999992895, 17.98437500000000000 ) ) ;
#12368=CARTESIAN_POINT ( 'NONE',  ( 1.799775606325937360E-14, -10.25000000000000000, 16.03125000000000000 ) ) ;
#12376=CARTESIAN_POINT ( 'NONE',  ( -1.929879867024197893E-14, -3.750000000000000000, 22.90625000000000355 ) ) ;
#12422=CARTESIAN_POINT ( 'NONE',  ( -1.929879867024197893E-14, -3.750000000000000000, 21.65625000000000355 ) ) ;
#12452=CARTESIAN_POINT ( 'NONE',  ( -3.749999999999996447, -7.561099074964554134, 24.84188170625848713 ) ) ;
#12466=CARTESIAN_POINT ( 'NONE',  ( 2.694853999681214862, -10.10844685921789043, 26.87313170625849423 ) ) ;
#12475=CARTESIAN_POINT ( 'NONE',  ( -3.724691934501248802, -5.885600066136383646, 16.67374329374151998 ) ) ;
#12483=CARTESIAN_POINT ( 'NONE',  ( -2.694853999681181556, -10.10844685921792241, 17.68936829374151287 ) ) ;
#12561=DIRECTION ( 'NONE',  ( -0.7057856980126717694, -0.7057856980126787638, -0.06109907496453172160 ) ) ;
#12566=CARTESIAN_POINT ( 'NONE',  ( 2.651650429449539104, -4.848349570550432475, 24.31250000000000000 ) ) ;
#12577=CARTESIAN_POINT ( 'NONE',  ( -1.929879867024197893E-14, -3.750000000000000000, 22.90625000000000355 ) ) ;
#12593=CARTESIAN_POINT ( 'NONE',  ( -2.749999999999999112, -7.438900925035484057, 16.59561829374151287 ) ) ;
#12600=CARTESIAN_POINT ( 'NONE',  ( 1.944543648263018731, -9.444543648262994751, 22.12500000000000000 ) ) ;
#12693=CARTESIAN_POINT ( 'NONE',  ( 1.901340078031373171, -9.487747218494639867, 19.87686829374151287 ) ) ;
#12797=CARTESIAN_POINT ( 'NONE',  ( 2.750000000000008438, -8.639087296525996607, 17.04687500000000000 ) ) ;
#12805=CARTESIAN_POINT ( 'NONE',  ( 2.750000000000008438, -8.639087296525996607, 19.54687499999999645 ) ) ;
#12812=CARTESIAN_POINT ( 'NONE',  ( -1.553300858899081538, -11.25000000000000711, 24.85937500000001421 ) ) ;
#12861=CARTESIAN_POINT ( 'NONE',  ( 1.553300858899086867, -3.749999999999992006, 19.23437500000000000 ) ) ;
#12890=CARTESIAN_POINT ( 'NONE',  ( -0.06109907496454585613, -4.750000000000000000, 20.15438170625849068 ) ) ;
#12904=CARTESIAN_POINT ( 'NONE',  ( 2.775308065498768517, -8.577988221561467341, 19.29500670625849068 ) ) ;
#12913=CARTESIAN_POINT ( 'NONE',  ( 3.775308065498752086, -6.007798216065404873, 15.89249329374151820 ) ) ;
#12921=CARTESIAN_POINT ( 'NONE',  ( 2.608446859217924629, -10.19485399968118422, 17.37686829374151287 ) ) ;
#12973=( GEOMETRIC_REPRESENTATION_CONTEXT ( 3 ) GLOBAL_UNCERTAINTY_ASSIGNED_CONTEXT ( ( #69912 ) ) GLOBAL_UNIT_ASSIGNED_CONTEXT ( ( #73083, #38862, #32535 ) ) REPRESENTATION_CONTEXT ( 'NONE', 'WORKASPACE' ) );
#13008=CARTESIAN_POINT ( 'NONE',  ( -2.651650429449535551, -10.15165042944956753, 26.18750000000000355 ) ) ;
#13016=CARTESIAN_POINT ( 'NONE',  ( -2.651650429449565305, -4.848349570550461785, 24.00000000000000000 ) ) ;
#13031=CARTESIAN_POINT ( 'NONE',  ( -1.200186371490524317, -10.22469193450124791, 17.61124329374151642 ) ) ;
#13040=CARTESIAN_POINT ( 'NONE',  ( -2.750000000000006217, -6.360912703474006946, 25.17187500000000000 ) ) ;
#13138=CARTESIAN_POINT ( 'NONE',  ( 2.750000000000002665, -7.561099074964516831, 22.22061829374151287 ) ) ;
#13244=CARTESIAN_POINT ( 'NONE',  ( -2.749999999999998224, -7.500000000000015987, 17.59375000000000000 ) ) ;
#13252=CARTESIAN_POINT ( 'NONE',  ( 1.944543648263018731, -9.444543648262994751, 20.87500000000000000 ) ) ;
#13307=CARTESIAN_POINT ( 'NONE',  ( -3.749999999999988454, -9.053300858899127945, 21.26562500000000000 ) ) ;
#13336=CARTESIAN_POINT ( 'NONE',  ( 1.200186371490561621, -10.22469193450123193, 19.45125670625849068 ) ) ;
#13349=CARTESIAN_POINT ( 'NONE',  ( 2.775308065498768517, -8.577988221561467341, 18.04500670625848713 ) ) ;
#13357=CARTESIAN_POINT ( 'NONE',  ( -1.492201783934593573, -3.724691934501250135, 23.07999329374151998 ) ) ;
#13362=CARTESIAN_POINT ( 'NONE',  ( -2.694853999681181556, -10.10844685921792241, 25.18936829374151642 ) ) ;
#13444=CARTESIAN_POINT ( 'NONE',  ( 2.320192649118979489E-14, -11.25000000000000000, 24.78125000000000000 ) ) ;
#13452=CARTESIAN_POINT ( 'NONE',  ( -2.694853999681210865, -4.891553140782108677, 14.99813170625848713 ) ) ;
#13471=CARTESIAN_POINT ( 'NONE',  ( 0.06109907496451789238, -4.749999999999998224, 19.40811829374151287 ) ) ;
#13480=CARTESIAN_POINT ( 'NONE',  ( 2.750000000000001776, -7.499999999999984013, 23.21875000000000000 ) ) ;
#13574=CARTESIAN_POINT ( 'NONE',  ( 2.775308065498755195, -6.422011778438505125, 22.14249329374151998 ) ) ;
#13680=CARTESIAN_POINT ( 'NONE',  ( -1.139087296525992166, -10.25000000000000533, 21.10937500000000711 ) ) ;
#13690=CARTESIAN_POINT ( 'NONE',  ( 1.799775606325937360E-14, -10.25000000000000000, 22.28125000000000355 ) ) ;
#13698=CARTESIAN_POINT ( 'NONE',  ( -2.651650429449535551, -10.15165042944956753, 26.18750000000000355 ) ) ;
#13748=CARTESIAN_POINT ( 'NONE',  ( 2.320192649118979489E-14, -11.25000000000000000, 18.53125000000000000 ) ) ;
#13776=CARTESIAN_POINT ( 'NONE',  ( 1.987747218494664292, -9.401340078031346081, 18.12313170625849068 ) ) ;
#13790=CARTESIAN_POINT ( 'NONE',  ( 0.06109907496454976272, -10.25000000000000000, 17.02938170625848713 ) ) ;
#13799=CARTESIAN_POINT ( 'NONE',  ( 1.614399933863618797, -3.775308065498751198, 20.73624329374151287 ) ) ;
#13805=CARTESIAN_POINT ( 'NONE',  ( 0.06109907496451268821, -3.749999999999999556, 24.40811829374151642 ) ) ;
#13886=CARTESIAN_POINT ( 'NONE',  ( -3.749999999999988454, -9.053300858899127945, 25.01562500000000000 ) ) ;
#13896=CARTESIAN_POINT ( 'NONE',  ( -2.651650429449565305, -4.848349570550461785, 26.50000000000000355 ) ) ;
#13911=CARTESIAN_POINT ( 'NONE',  ( -2.749999999999999112, -7.438900925035484057, 20.34561829374151287 ) ) ;
#13918=CARTESIAN_POINT ( 'NONE',  ( -1.944543648262992530, -9.444543648263016067, 26.18750000000000355 ) ) ;
#14002=CARTESIAN_POINT ( 'NONE',  ( -1.553300858899081538, -11.25000000000000711, 14.85937500000000355 ) ) ;
#14017=CARTESIAN_POINT ( 'NONE',  ( -0.06109907496451398579, -10.25000000000000178, 18.78311829374151287 ) ) ;
#14123=CARTESIAN_POINT ( 'NONE',  ( -1.944543648263014957, -5.555456351737005249, 14.00000000000000178 ) ) ;
#14125=CARTESIAN_POINT ( 'NONE',  ( 1.139087296525997273, -4.749999999999992895, 16.73437500000000000 ) ) ;
#14134=CARTESIAN_POINT ( 'NONE',  ( -1.139087296525992166, -10.25000000000000533, 18.60937500000000355 ) ) ;
#14142=CARTESIAN_POINT ( 'NONE',  ( 2.320192649118979489E-14, -11.25000000000000000, 24.78125000000000000 ) ) ;
#14192=CARTESIAN_POINT ( 'NONE',  ( 3.749999999999992006, -5.946699141100872943, 21.89062500000000355 ) ) ;
#14226=CARTESIAN_POINT ( 'NONE',  ( -2.749999999999997780, -7.561099074964547917, 17.34188170625849068 ) ) ;
#14237=CARTESIAN_POINT ( 'NONE',  ( 0.06109907496454976272, -10.25000000000000000, 18.27938170625849068 ) ) ;
#14246=CARTESIAN_POINT ( 'NONE',  ( 0.06109907496451268821, -3.749999999999999556, 24.40811829374151642 ) ) ;
#14251=CARTESIAN_POINT ( 'NONE',  ( 2.651650429449569302, -10.15165042944953733, 14.62500000000000000 ) ) ;
#14332=CARTESIAN_POINT ( 'NONE',  ( 0.06109907496455496689, -11.24999999999999822, 17.02938170625848713 ) ) ;
#14341=CARTESIAN_POINT ( 'NONE',  ( 1.492201783934554493, -3.724691934501233703, 17.73250670625848713 ) ) ;
#14354=CARTESIAN_POINT ( 'NONE',  ( -2.775308065498752086, -8.577988221561495763, 21.51749329374151998 ) ) ;
#14407=EDGE_CURVE ( 'NONE', #76825, #55297, #36278, .T. ) ;
#14465=CARTESIAN_POINT ( 'NONE',  ( 2.694853999681185108, -4.891553140782077591, 14.56436829374151287 ) ) ;
#14567=CARTESIAN_POINT ( 'NONE',  ( -2.749999999999991562, -8.639087296526025028, 25.01562500000000000 ) ) ;
#14585=CARTESIAN_POINT ( 'NONE',  ( 3.749999999999992006, -5.946699141100872943, 25.64062500000000000 ) ) ;
#14638=CARTESIAN_POINT ( 'NONE',  ( -3.749999999999988454, -9.053300858899127945, 23.76562500000000000 ) ) ;
#14673=CARTESIAN_POINT ( 'NONE',  ( -2.775308065498764964, -6.422011778438537988, 16.17000670625848713 ) ) ;
#14684=CARTESIAN_POINT ( 'NONE',  ( -2.724691934501232371, -8.700186371490559623, 21.01375670625849068 ) ) ;
#14691=CARTESIAN_POINT ( 'NONE',  ( -3.749999999999997780, -7.438900925035489387, 25.34561829374151642 ) ) ;
#14696=CARTESIAN_POINT ( 'NONE',  ( 1.614399933863618797, -3.775308065498751198, 21.98624329374151642 ) ) ;
#14786=CARTESIAN_POINT ( 'NONE',  ( -1.553300858899125059, -3.750000000000009326, 25.32812500000000711 ) ) ;
#14795=CARTESIAN_POINT ( 'NONE',  ( -1.614399933863656544, -3.775308065498769405, 15.07625670625849068 ) ) ;
#14811=CARTESIAN_POINT ( 'NONE',  ( -1.077988221561493543, -4.724691934501247914, 20.57999329374151998 ) ) ;
#14917=CARTESIAN_POINT ( 'NONE',  ( -1.901340078031369618, -5.512252781505359245, 25.50186829374151287 ) ) ;
#15019=CARTESIAN_POINT ( 'NONE',  ( 1.944543648262996083, -5.555456351736983045, 23.06250000000000000 ) ) ;
#15119=CARTESIAN_POINT ( 'NONE',  ( -2.724691934501232371, -8.700186371490559623, 22.26375670625849068 ) ) ;
#15131=CARTESIAN_POINT ( 'NONE',  ( -2.775308065498764964, -6.422011778438537988, 23.67000670625849779 ) ) ;
#15139=CARTESIAN_POINT ( 'NONE',  ( 3.750000000000000888, -7.499999999999978684, 14.46875000000000000 ) ) ;
#15144=CARTESIAN_POINT ( 'NONE',  ( 2.694853999681185108, -4.891553140782077591, 24.56436829374151287 ) ) ;
#15228=CARTESIAN_POINT ( 'NONE',  ( 3.749999999999999556, -7.438900925035446754, 20.46688170625848713 ) ) ;
#15237=CARTESIAN_POINT ( 'NONE',  ( -2.608446859217889546, -10.19485399968121264, 17.18563170625848713 ) ) ;
#15252=CARTESIAN_POINT ( 'NONE',  ( -1.901340078031369618, -5.512252781505359245, 20.50186829374151287 ) ) ;
#15356=CARTESIAN_POINT ( 'NONE',  ( 2.750000000000002665, -7.561099074964516831, 23.47061829374151642 ) ) ;
#15465=CARTESIAN_POINT ( 'NONE',  ( 2.750000000000008438, -8.639087296525996607, 22.04687500000000000 ) ) ;
#15530=CARTESIAN_POINT ( 'NONE',  ( 3.749999999999992006, -5.946699141100872943, 23.14062499999999645 ) ) ;
#15562=CARTESIAN_POINT ( 'NONE',  ( -2.775308065498764964, -6.422011778438537988, 21.17000670625848713 ) ) ;
#15564=CARTESIAN_POINT ( 'NONE',  ( 0.07543784382008528189, -3.752057646953216530, 13.99999999999965894 ) ) ;
#15574=CARTESIAN_POINT ( 'NONE',  ( -2.724691934501232371, -8.700186371490559623, 22.26375670625849068 ) ) ;
#15581=CARTESIAN_POINT ( 'NONE',  ( -2.651650429449565305, -4.848349570550461785, 15.25000000000000000 ) ) ;
#15587=CARTESIAN_POINT ( 'NONE',  ( 2.320192649118979489E-14, -11.25000000000000000, 18.53125000000000000 ) ) ;
#15668=CARTESIAN_POINT ( 'NONE',  ( -0.06109907496455085213, -3.750000000000000888, 22.65438170625849068 ) ) ;
#15679=CARTESIAN_POINT ( 'NONE',  ( 2.608446859217893099, -4.805146000318787358, 19.06063170625849068 ) ) ;
#15694=CARTESIAN_POINT ( 'NONE',  ( 2.694853999681185108, -4.891553140782077591, 14.56436829374151287 ) ) ;
#15776=CARTESIAN_POINT ( 'NONE',  ( -3.749999999999997335, -7.500000000000021316, 16.34375000000000000 ) ) ;
#15787=CARTESIAN_POINT ( 'NONE',  ( -1.553300858899125059, -3.750000000000009326, 15.32812500000000355 ) ) ;
#15802=CARTESIAN_POINT ( 'NONE',  ( -3.775308065498748977, -8.992201783934593351, 14.01749329374151642 ) ) ;
#15806=CARTESIAN_POINT ( 'NONE',  ( -1.139087296526025916, -4.750000000000006217, 21.57812500000000355 ) ) ;
#15812=CARTESIAN_POINT ( 'NONE',  ( -1.409462824231155764E-14, -4.749999999999999112, 15.40625000000000000 ) ) ;
#15908=CARTESIAN_POINT ( 'NONE',  ( 2.750000000000008438, -8.639087296525996607, 24.54687500000000000 ) ) ;
#16005=CARTESIAN_POINT ( 'NONE',  ( -1.077988221561460236, -10.27530806549876452, 24.60750670625849779 ) ) ;
#16007=CARTESIAN_POINT ( 'NONE',  ( 3.181675156714246278, -8.024245293229201437, 13.99999999999999289 ) ) ;
#16014=CARTESIAN_POINT ( 'NONE',  ( -1.987747218494660295, -5.598659921968651254, 21.24813170625848713 ) ) ;
#16022=CARTESIAN_POINT ( 'NONE',  ( 1.553300858899087311, -3.749999999999992006, 16.73437500000000000 ) ) ;
#16027=CARTESIAN_POINT ( 'NONE',  ( -3.749999999999997335, -7.500000000000021316, 17.59375000000000000 ) ) ;
#16029=PLANE ( 'NONE',  #20272 ) ;
#16065=CARTESIAN_POINT ( 'NONE',  ( 3.749999999999992006, -5.946699141100872943, 20.64062500000000000 ) ) ;
#16105=CARTESIAN_POINT ( 'NONE',  ( 3.775308065498768517, -8.992201783934554271, 20.54500670625849068 ) ) ;
#16114=CARTESIAN_POINT ( 'NONE',  ( -0.06109907496455085213, -3.750000000000000888, 22.65438170625849068 ) ) ;
#16128=CARTESIAN_POINT ( 'NONE',  ( -0.06109907496450878162, -11.25000000000000000, 13.78311829374151287 ) ) ;
#16209=CARTESIAN_POINT ( 'NONE',  ( -3.750000000000008438, -5.946699141100917352, 16.42187500000000000 ) ) ;
#16219=CARTESIAN_POINT ( 'NONE',  ( 1.553300858899087311, -3.749999999999992006, 15.48437500000000178 ) ) ;
#16232=CARTESIAN_POINT ( 'NONE',  ( -3.775308065498748977, -8.992201783934593351, 15.26749329374151465 ) ) ;
#16237=CARTESIAN_POINT ( 'NONE',  ( -2.750000000000007105, -6.360912703474006946, 25.17187500000000000 ) ) ;
#16340=CARTESIAN_POINT ( 'NONE',  ( -1.409462824231155764E-14, -4.749999999999999112, 21.65625000000000355 ) ) ;
#16371=DIRECTION ( 'NONE',  ( 0.7057856980126718804, 0.7057856980126787638, 0.06109907496453181874 ) ) ;
#16407=CARTESIAN_POINT ( 'NONE',  ( -2.651650429449535551, -10.15165042944956753, 24.93750000000000000 ) ) ;
#16443=CARTESIAN_POINT ( 'NONE',  ( -0.06109907496454585613, -4.750000000000000000, 25.15438170625849068 ) ) ;
#16445=CARTESIAN_POINT ( 'NONE',  ( 3.174020486757124004, -8.011881170783730965, 14.00000000000000888 ) ) ;
#16452=CARTESIAN_POINT ( 'NONE',  ( 2.775308065498768517, -8.577988221561467341, 24.29500670625849423 ) ) ;
#16462=CARTESIAN_POINT ( 'NONE',  ( -1.553300858899081538, -11.25000000000000711, 16.10937500000000355 ) ) ;
#16468=CARTESIAN_POINT ( 'NONE',  ( -1.553300858899125059, -3.750000000000009326, 15.32812500000000355 ) ) ;
#16503=CARTESIAN_POINT ( 'NONE',  ( 1.553300858899129944, -11.24999999999998934, 22.20312500000000000 ) ) ;
#16541=CARTESIAN_POINT ( 'NONE',  ( 2.694853999681214862, -10.10844685921789043, 18.12313170625849068 ) ) ;
#16550=CARTESIAN_POINT ( 'NONE',  ( 3.749999999999999556, -7.438900925035446754, 21.71688170625848713 ) ) ;
#16564=CARTESIAN_POINT ( 'NONE',  ( -1.492201783934593573, -3.724691934501250135, 15.57999329374151110 ) ) ;
#16642=CARTESIAN_POINT ( 'NONE',  ( -2.651650429449535551, -10.15165042944956753, 18.68750000000000000 ) ) ;
#16651=CARTESIAN_POINT ( 'NONE',  ( -1.929879867024197893E-14, -3.750000000000000000, 17.90625000000000000 ) ) ;
#16667=CARTESIAN_POINT ( 'NONE',  ( -3.749999999999997780, -7.438900925035489387, 17.84561829374150932 ) ) ;
#16672=CARTESIAN_POINT ( 'NONE',  ( -1.944543648263014957, -5.555456351737005249, 25.25000000000000000 ) ) ;
#16680=CARTESIAN_POINT ( 'NONE',  ( 1.799775606325937360E-14, -10.25000000000000000, 18.53125000000000000 ) ) ;
#16773=CARTESIAN_POINT ( 'NONE',  ( -2.775308065498752086, -8.577988221561495763, 16.51749329374151642 ) ) ;
#16883=CARTESIAN_POINT ( 'NONE',  ( -2.724691934501232371, -8.700186371490559623, 23.51375670625848713 ) ) ;
#16885=CARTESIAN_POINT ( 'NONE',  ( 3.064640908609403969, -5.597845033694389016, 14.00000000000009059 ) ) ;
#16895=CARTESIAN_POINT ( 'NONE',  ( 1.077988221561464899, -4.724691934501233703, 21.48250670625849068 ) ) ;
#16904=CARTESIAN_POINT ( 'NONE',  ( 3.749999999999992006, -5.946699141100872943, 16.89062500000000000 ) ) ;
#16910=CARTESIAN_POINT ( 'NONE',  ( -1.929879867024197893E-14, -3.750000000000000000, 15.40625000000000000 ) ) ;
#16948=CARTESIAN_POINT ( 'NONE',  ( -3.750000000000008438, -5.946699141100917352, 20.17187500000000000 ) ) ;
#16988=CARTESIAN_POINT ( 'NONE',  ( 2.608446859217893099, -4.805146000318787358, 17.81063170625849068 ) ) ;
#16998=CARTESIAN_POINT ( 'NONE',  ( -1.614399933863656544, -3.775308065498769405, 20.07625670625849068 ) ) ;
#17012=CARTESIAN_POINT ( 'NONE',  ( 1.614399933863618797, -3.775308065498751198, 15.73624329374151998 ) ) ;
#17091=CARTESIAN_POINT ( 'NONE',  ( -1.929879867024197893E-14, -3.750000000000000000, 19.15625000000000000 ) ) ;
#17100=CARTESIAN_POINT ( 'NONE',  ( 2.320192649118979489E-14, -11.25000000000000000, 16.03125000000000000 ) ) ;
#17113=CARTESIAN_POINT ( 'NONE',  ( -2.608446859217920633, -4.805146000318815780, 16.75186829374151287 ) ) ;
#17119=CARTESIAN_POINT ( 'NONE',  ( 2.749999999999995115, -6.360912703473971419, 23.14062500000000000 ) ) ;
#17123=CARTESIAN_POINT ( 'NONE',  ( 1.139087296525997051, -4.749999999999992895, 20.48437500000000000 ) ) ;
#17220=CARTESIAN_POINT ( 'NONE',  ( -0.06109907496451398579, -10.25000000000000178, 13.78311829374151287 ) ) ;
#17331=CARTESIAN_POINT ( 'NONE',  ( -2.750000000000007105, -6.360912703474006946, 15.17187500000000000 ) ) ;
#17341=CARTESIAN_POINT ( 'NONE',  ( -2.750000000000007105, -6.360912703474006946, 16.42187500000000000 ) ) ;
#17352=CARTESIAN_POINT ( 'NONE',  ( -1.553300858899081538, -11.25000000000000711, 23.60937500000000711 ) ) ;
#17396=CARTESIAN_POINT ( 'NONE',  ( 2.651650429449569302, -10.15165042944953733, 19.62500000000000000 ) ) ;
#17405=CARTESIAN_POINT ( 'NONE',  ( -2.651650429449535551, -10.15165042944956753, 17.43750000000000000 ) ) ;
#17438=CARTESIAN_POINT ( 'NONE',  ( 0.06109907496455496689, -11.24999999999999822, 25.77938170625848713 ) ) ;
#17447=CARTESIAN_POINT ( 'NONE',  ( 2.694853999681214862, -10.10844685921789043, 23.12313170625848713 ) ) ;
#17461=CARTESIAN_POINT ( 'NONE',  ( -1.492201783934593573, -3.724691934501250135, 14.32999329374151465 ) ) ;
#17544=CARTESIAN_POINT ( 'NONE',  ( 3.749999999999992006, -5.946699141100872943, 15.64062500000000178 ) ) ;
#17554=CARTESIAN_POINT ( 'NONE',  ( -3.749999999999988454, -9.053300858899127945, 17.51562500000000000 ) ) ;
#17571=CARTESIAN_POINT ( 'NONE',  ( 1.492201783934598236, -11.27530806549875031, 19.95499329374151642 ) ) ;
#17576=CARTESIAN_POINT ( 'NONE',  ( 1.901340078031373171, -9.487747218494639867, 13.62686829374151642 ) ) ;
#17582=CARTESIAN_POINT ( 'NONE',  ( -1.139087296526025250, -4.750000000000006217, 19.07812500000000000 ) ) ;
#17676=CARTESIAN_POINT ( 'NONE',  ( 1.987747218494642309, -5.598659921968629050, 15.81436829374151465 ) ) ;
#17709=DIRECTION ( 'NONE',  ( 0.7057856980126718804, 0.7057856980126787638, 0.06109907496453181874 ) ) ;
#17787=CARTESIAN_POINT ( 'NONE',  ( 2.724691934501235036, -6.299813628509441266, 26.63875670625848713 ) ) ;
#17797=CARTESIAN_POINT ( 'NONE',  ( -1.409462824231155764E-14, -4.749999999999999112, 14.15625000000000000 ) ) ;
#17805=CARTESIAN_POINT ( 'NONE',  ( -1.553300858899081538, -11.25000000000000711, 22.35937500000000711 ) ) ;
#17847=CARTESIAN_POINT ( 'NONE',  ( 2.651650429449539104, -4.848349570550432475, 21.81250000000000000 ) ) ;
#17854=CARTESIAN_POINT ( 'NONE',  ( 1.553300858899086867, -3.749999999999992006, 14.23437500000000178 ) ) ;
#17885=CARTESIAN_POINT ( 'NONE',  ( -3.775308065498766297, -6.007798216065450170, 26.17000670625849068 ) ) ;
#17893=CARTESIAN_POINT ( 'NONE',  ( 1.077988221561464899, -4.724691934501233703, 15.23250670625848713 ) ) ;
#17906=CARTESIAN_POINT ( 'NONE',  ( -1.492201783934593573, -3.724691934501250135, 16.82999329374151287 ) ) ;
#17993=CARTESIAN_POINT ( 'NONE',  ( 3.750000000000000888, -7.499999999999978684, 21.96875000000000355 ) ) ;
#18001=CARTESIAN_POINT ( 'NONE',  ( 2.651650429449539104, -4.848349570550432475, 20.56250000000000000 ) ) ;
#18020=CARTESIAN_POINT ( 'NONE',  ( -1.139087296525992166, -10.25000000000000533, 23.60937500000000711 ) ) ;
#18026=CARTESIAN_POINT ( 'NONE',  ( -1.944543648262992530, -9.444543648263016067, 21.18750000000000000 ) ) ;
#18049=DIRECTION ( 'NONE',  ( -0.7057856980126717694, -0.7057856980126787638, -0.06109907496453172160 ) ) ;
#18121=CARTESIAN_POINT ( 'NONE',  ( 1.901340078031373171, -9.487747218494639867, 17.37686829374151287 ) ) ;
#18229=CARTESIAN_POINT ( 'NONE',  ( -1.139087296525992166, -10.25000000000000533, 16.10937500000000355 ) ) ;
#18238=CARTESIAN_POINT ( 'NONE',  ( -1.944543648262992530, -9.444543648263016067, 14.93750000000000000 ) ) ;
#18246=CARTESIAN_POINT ( 'NONE',  ( 3.749999999999992006, -5.946699141100872943, 23.14062500000000000 ) ) ;
#18286=CARTESIAN_POINT ( 'NONE',  ( 1.553300858899087311, -3.749999999999992006, 25.48437500000000000 ) ) ;
#18291=CARTESIAN_POINT ( 'NONE',  ( -3.749999999999997335, -7.500000000000021316, 17.59375000000000000 ) ) ;
#18326=CARTESIAN_POINT ( 'NONE',  ( -1.492201783934549164, -11.27530806549876807, 24.60750670625849779 ) ) ;
#18335=CARTESIAN_POINT ( 'NONE',  ( 0.06109907496454976272, -10.25000000000000000, 15.77938170625848890 ) ) ;
#18352=CARTESIAN_POINT ( 'NONE',  ( 0.06109907496451268821, -3.749999999999999556, 20.65811829374151287 ) ) ;
#18435=CARTESIAN_POINT ( 'NONE',  ( -1.929879867024197893E-14, -3.750000000000000000, 22.90625000000000355 ) ) ;
#18440=EDGE_CURVE ( 'NONE', #28286, #58074, #454, .T. ) ;
#18446=CARTESIAN_POINT ( 'NONE',  ( -1.553300858899125059, -3.750000000000009326, 21.57812500000000355 ) ) ;
#18465=CARTESIAN_POINT ( 'NONE',  ( 1.200186371490529202, -4.775308065498752974, 18.23624329374151642 ) ) ;
#18471=CARTESIAN_POINT ( 'NONE',  ( -1.139087296525992388, -10.25000000000000711, 17.35937499999999645 ) ) ;
#18564=CARTESIAN_POINT ( 'NONE',  ( 1.200186371490529202, -4.775308065498752974, 14.48624329374151465 ) ) ;
#18591=SURFACE_STYLE_FILL_AREA ( #23995 ) ;
#18678=CARTESIAN_POINT ( 'NONE',  ( -1.944543648262992530, -9.444543648263016067, 16.18750000000000000 ) ) ;
#18688=CARTESIAN_POINT ( 'NONE',  ( -2.750000000000007105, -6.360912703474006946, 15.17187500000000000 ) ) ;
#18696=CARTESIAN_POINT ( 'NONE',  ( -2.651650429449565305, -4.848349570550461785, 19.00000000000000000 ) ) ;
#18742=CARTESIAN_POINT ( 'NONE',  ( -3.749999999999997335, -7.500000000000021316, 15.09375000000000000 ) ) ;
#18773=CARTESIAN_POINT ( 'NONE',  ( -2.608446859217889546, -10.19485399968121264, 27.18563170625849068 ) ) ;
#18784=CARTESIAN_POINT ( 'NONE',  ( 2.608446859217893099, -4.805146000318787358, 24.06063170625849423 ) ) ;
#18798=CARTESIAN_POINT ( 'NONE',  ( -1.614399933863613468, -11.22469193450124969, 18.86124329374151287 ) ) ;
#18875=CARTESIAN_POINT ( 'NONE',  ( 1.553300858899087311, -3.749999999999992006, 20.48437500000000000 ) ) ;
#18887=CARTESIAN_POINT ( 'NONE',  ( 3.750000000000000888, -7.499999999999978684, 23.21875000000000000 ) ) ;
#18904=CARTESIAN_POINT ( 'NONE',  ( 1.077988221561497539, -10.27530806549875386, 16.20499329374151642 ) ) ;
#18910=CARTESIAN_POINT ( 'NONE',  ( -2.750000000000006217, -6.360912703474006946, 22.67187499999999645 ) ) ;
#19006=CARTESIAN_POINT ( 'NONE',  ( -2.775308065498752086, -8.577988221561495763, 20.26749329374151998 ) ) ;
#19093=CARTESIAN_POINT ( 'NONE',  ( -2.115085314324983479, -5.372444627205700485, 13.85595217397070478 ) ) ;
#19116=CARTESIAN_POINT ( 'NONE',  ( 1.200186371490561621, -10.22469193450123193, 26.95125670625849068 ) ) ;
#19124=CARTESIAN_POINT ( 'NONE',  ( 2.750000000000008438, -8.639087296525996607, 14.54687500000000178 ) ) ;
#19131=CARTESIAN_POINT ( 'NONE',  ( -1.553300858899125059, -3.750000000000009326, 22.82812500000000355 ) ) ;
#19180=CARTESIAN_POINT ( 'NONE',  ( -2.651650429449565305, -4.848349570550461785, 15.25000000000000000 ) ) ;
#19195=CARTESIAN_POINT ( 'NONE',  ( -1.216139819124259613, -4.489159616049914980, 13.64598852175840626 ) ) ;
#19214=CARTESIAN_POINT ( 'NONE',  ( -3.724691934501229262, -9.114399933863657211, 24.76375670625848713 ) ) ;
#19227=CARTESIAN_POINT ( 'NONE',  ( -1.614399933863656544, -3.775308065498769405, 25.07625670625849423 ) ) ;
#19236=CARTESIAN_POINT ( 'NONE',  ( -3.749999999999997780, -7.438900925035489387, 19.09561829374150932 ) ) ;
#19242=CARTESIAN_POINT ( 'NONE',  ( 3.750000000000001776, -7.561099074964511502, 18.47061829374151287 ) ) ;
#19323=CARTESIAN_POINT ( 'NONE',  ( -1.929879867024197893E-14, -3.750000000000000000, 21.65625000000000355 ) ) ;
#19333=CARTESIAN_POINT ( 'NONE',  ( 2.651650429449569302, -10.15165042944953733, 20.87500000000000000 ) ) ;
#19348=CARTESIAN_POINT ( 'NONE',  ( -0.06109907496451398579, -10.25000000000000178, 17.53311829374151287 ) ) ;
#19353=CARTESIAN_POINT ( 'NONE',  ( -1.409462824231155764E-14, -4.749999999999999112, 22.90625000000000355 ) ) ;
#19447=CARTESIAN_POINT ( 'NONE',  ( 1.200186371490529202, -4.775308065498752974, 20.73624329374151287 ) ) ;
#19551=CARTESIAN_POINT ( 'NONE',  ( 2.750000000000008438, -8.639087296525996607, 20.79687500000000000 ) ) ;
#19560=CARTESIAN_POINT ( 'NONE',  ( -1.409462824231155764E-14, -4.749999999999999112, 20.40625000000000000 ) ) ;
#19617=CARTESIAN_POINT ( 'NONE',  ( -1.553300858899081760, -11.25000000000000888, 19.85937500000000711 ) ) ;
#19650=CARTESIAN_POINT ( 'NONE',  ( 1.987747218494664292, -9.401340078031346081, 16.87313170625849068 ) ) ;
#19663=CARTESIAN_POINT ( 'NONE',  ( -3.749999999999996447, -7.561099074964554134, 26.09188170625848358 ) ) ;
#19670=CARTESIAN_POINT ( 'NONE',  ( -1.492201783934593573, -3.724691934501250135, 19.32999329374151642 ) ) ;
#19677=CARTESIAN_POINT ( 'NONE',  ( -3.749999999999997780, -7.438900925035489387, 20.34561829374151287 ) ) ;
#19765=CARTESIAN_POINT ( 'NONE',  ( 3.750000000000009770, -9.053300858899081760, 20.79687500000000000 ) ) ;
#19774=CARTESIAN_POINT ( 'NONE',  ( -1.553300858899125059, -3.750000000000009326, 22.82812500000000355 ) ) ;
#19788=CARTESIAN_POINT ( 'NONE',  ( -1.987747218494638313, -9.401340078031370950, 16.43936829374151287 ) ) ;
#19796=CARTESIAN_POINT ( 'NONE',  ( 1.139087296525997051, -4.749999999999992895, 24.23437500000000355 ) ) ;
#19887=CARTESIAN_POINT ( 'NONE',  ( -2.724691934501246582, -6.299813628509474128, 19.17374329374151642 ) ) ;
#19917=CLOSED_SHELL ( 'NONE', ( #28910, #86761, #83372, #11512, #19975, #1738 ) ) ;
#19975=ADVANCED_FACE ( 'NONE', ( #20598 ), #48062, .T. ) ;
#19986=COLOUR_RGB ( '', 0.66274510, 0.83137255, 0.94901961) ;
#19992=CARTESIAN_POINT ( 'NONE',  ( 1.139087296526029469, -10.24999999999999467, 17.20312500000000000 ) ) ;
#20002=CARTESIAN_POINT ( 'NONE',  ( -1.139087296526025916, -4.750000000000006217, 20.32812500000000000 ) ) ;
#20064=CARTESIAN_POINT ( 'NONE',  ( -1.553300858899125059, -3.750000000000009326, 20.32812500000000711 ) ) ;
#20096=CARTESIAN_POINT ( 'NONE',  ( -1.200186371490556958, -4.775308065498765409, 16.32625670625849068 ) ) ;
#20110=CARTESIAN_POINT ( 'NONE',  ( 1.901340078031349856, -5.512252781505337929, 20.31063170625848713 ) ) ;
#20122=CARTESIAN_POINT ( 'NONE',  ( -3.749999999999997780, -7.438900925035489387, 21.59561829374151287 ) ) ;
#20126=CARTESIAN_POINT ( 'NONE',  ( 1.492201783934598236, -11.27530806549875031, 24.95499329374151287 ) ) ;
#20153=CARTESIAN_POINT ( 'NONE',  ( -2.651650429449565305, -4.848349570550461785, 26.50000000000000355 ) ) ;
#20212=CARTESIAN_POINT ( 'NONE',  ( 2.651650429449569302, -10.15165042944953733, 24.62500000000000000 ) ) ;
#20220=CARTESIAN_POINT ( 'NONE',  ( 2.608446859217893099, -4.805146000318787358, 17.81063170625849068 ) ) ;
#20236=CARTESIAN_POINT ( 'NONE',  ( -2.724691934501246582, -6.299813628509474128, 14.17374329374151287 ) ) ;
#20244=CARTESIAN_POINT ( 'NONE',  ( -2.749999999999998224, -7.500000000000015987, 21.34375000000000000 ) ) ;
#20272=AXIS2_PLACEMENT_3D ( 'NONE', #50234, #78168, #70529 ) ;
#20343=CARTESIAN_POINT ( 'NONE',  ( -1.987747218494638313, -9.401340078031370950, 21.43936829374151642 ) ) ;
#20395=CARTESIAN_POINT ( 'NONE',  ( 3.750000000000009770, -9.053300858899081760, 24.54687500000000000 ) ) ;
#20444=CARTESIAN_POINT ( 'NONE',  ( -1.944543648262992530, -9.444543648263016067, 17.43750000000000000 ) ) ;
#20453=CARTESIAN_POINT ( 'NONE',  ( 2.750000000000001776, -7.499999999999984013, 21.96875000000000355 ) ) ;
#20506=CARTESIAN_POINT ( 'NONE',  ( 2.651650429449569302, -10.15165042944953733, 18.37500000000000355 ) ) ;
#20536=CARTESIAN_POINT ( 'NONE',  ( 2.724691934501235036, -6.299813628509441266, 15.38875670625848890 ) ) ;
#20550=CARTESIAN_POINT ( 'NONE',  ( 2.775308065498768517, -8.577988221561467341, 20.54500670625849068 ) ) ;
#20557=CARTESIAN_POINT ( 'NONE',  ( 2.694853999681185108, -4.891553140782077591, 23.31436829374150932 ) ) ;
#20562=CARTESIAN_POINT ( 'NONE',  ( 2.608446859217924629, -10.19485399968118422, 22.37686829374150932 ) ) ;
#20598=FACE_OUTER_BOUND ( 'NONE', #71824, .T. ) ;
#20643=CARTESIAN_POINT ( 'NONE',  ( -3.749999999999988454, -9.053300858899127945, 26.26562500000000000 ) ) ;
#20654=CARTESIAN_POINT ( 'NONE',  ( 3.750000000000009770, -9.053300858899081760, 25.79687500000000355 ) ) ;
#20669=CARTESIAN_POINT ( 'NONE',  ( -2.749999999999999112, -7.438900925035484057, 21.59561829374151287 ) ) ;
#20678=CARTESIAN_POINT ( 'NONE',  ( 1.139087296526029469, -10.24999999999999289, 25.95312500000000000 ) ) ;
#20758=CARTESIAN_POINT ( 'NONE',  ( -1.929879867024197893E-14, -3.750000000000000000, 14.15625000000000000 ) ) ;
#20774=CARTESIAN_POINT ( 'NONE',  ( 0.06109907496451789238, -4.749999999999998224, 18.15811829374151642 ) ) ;
#20779=FILL_AREA_STYLE_COLOUR ( '', #19986 ) ;
#20830=CARTESIAN_POINT ( 'NONE',  ( -3.749999999999997335, -7.500000000000021316, 26.34375000000000000 ) ) ;
#20876=CARTESIAN_POINT ( 'NONE',  ( -2.750000000000007105, -6.360912703474006946, 21.42187500000000000 ) ) ;
#20884=CARTESIAN_POINT ( 'NONE',  ( -2.749999999999991562, -8.639087296526025028, 18.76562500000000000 ) ) ;
#20942=CARTESIAN_POINT ( 'NONE',  ( 2.651650429449569302, -10.15165042944953733, 20.87500000000000000 ) ) ;
#20968=CARTESIAN_POINT ( 'NONE',  ( -1.987747218494660295, -5.598659921968651254, 18.74813170625849068 ) ) ;
#20981=CARTESIAN_POINT ( 'NONE',  ( -0.06109907496454585613, -4.750000000000000000, 18.90438170625848713 ) ) ;
#20989=CARTESIAN_POINT ( 'NONE',  ( -2.694853999681181556, -10.10844685921792241, 21.43936829374151642 ) ) ;
#20994=CARTESIAN_POINT ( 'NONE',  ( 1.492201783934598236, -11.27530806549875031, 22.45499329374151287 ) ) ;
#21060=CARTESIAN_POINT ( 'NONE',  ( -1.944543648263015179, -5.555456351737005249, 26.50000000000000355 ) ) ;
#21078=CARTESIAN_POINT ( 'NONE',  ( 2.608446859217893099, -4.805146000318787358, 16.56063170625848713 ) ) ;
#21086=CARTESIAN_POINT ( 'NONE',  ( -3.749999999999996447, -7.561099074964554134, 18.59188170625849068 ) ) ;
#21102=CARTESIAN_POINT ( 'NONE',  ( -2.775308065498752086, -8.577988221561495763, 20.26749329374151998 ) ) ;
#21199=CARTESIAN_POINT ( 'NONE',  ( -3.750000000000008438, -5.946699141100917352, 15.17187500000000000 ) ) ;
#21214=CARTESIAN_POINT ( 'NONE',  ( 3.775308065498752086, -6.007798216065404873, 13.39249329374151642 ) ) ;
#21222=CARTESIAN_POINT ( 'NONE',  ( 2.750000000000001776, -7.499999999999984013, 14.46875000000000000 ) ) ;
#21267=CARTESIAN_POINT ( 'NONE',  ( 2.651650429449569302, -10.15165042944953733, 24.62500000000000000 ) ) ;
#21319=CARTESIAN_POINT ( 'NONE',  ( 2.750000000000008438, -8.639087296525996607, 18.29687500000000000 ) ) ;
#21339=CARTESIAN_POINT ( 'NONE',  ( 2.651650429449569302, -10.15165042944953733, 24.62500000000000000 ) ) ;
#21394=CARTESIAN_POINT ( 'NONE',  ( -1.553300858899125059, -3.750000000000009326, 24.07812500000000711 ) ) ;
#21426=CARTESIAN_POINT ( 'NONE',  ( -2.749999999999997780, -7.561099074964547917, 19.84188170625848713 ) ) ;
#21436=CARTESIAN_POINT ( 'NONE',  ( -2.775308065498764964, -6.422011778438537988, 17.42000670625848713 ) ) ;
#21444=CARTESIAN_POINT ( 'NONE',  ( 3.775308065498752086, -6.007798216065404873, 22.14249329374151998 ) ) ;
#21451=CARTESIAN_POINT ( 'NONE',  ( 3.750000000000001776, -7.561099074964511502, 23.47061829374151642 ) ) ;
#21503=AXIS2_PLACEMENT_3D ( 'NONE', #11226, #12561, #38695 ) ;
#21531=CARTESIAN_POINT ( 'NONE',  ( -1.614399933863656544, -3.775308065498769405, 17.57625670625849068 ) ) ;
#21539=CARTESIAN_POINT ( 'NONE',  ( 3.749999999999999556, -7.438900925035446754, 16.71688170625848713 ) ) ;
#21555=CARTESIAN_POINT ( 'NONE',  ( 1.077988221561497539, -10.27530806549875386, 23.70499329374151642 ) ) ;
#21662=CARTESIAN_POINT ( 'NONE',  ( 1.077988221561497539, -10.27530806549875386, 23.70499329374151642 ) ) ;
#21672=CARTESIAN_POINT ( 'NONE',  ( -2.750000000000006217, -6.360912703474006946, 15.17187500000000000 ) ) ;
#21768=CARTESIAN_POINT ( 'NONE',  ( -2.750000000000007105, -6.360912703474006946, 23.92187500000000355 ) ) ;
#21839=CARTESIAN_POINT ( 'NONE',  ( 3.750000000000009770, -9.053300858899081760, 24.54687500000000000 ) ) ;
#21864=FACE_OUTER_BOUND ( 'NONE', #26755, .T. ) ;
#21869=CARTESIAN_POINT ( 'NONE',  ( 2.775308065498768517, -8.577988221561467341, 23.04500670625849068 ) ) ;
#21881=CARTESIAN_POINT ( 'NONE',  ( 2.724691934501235036, -6.299813628509441266, 17.88875670625848713 ) ) ;
#21889=CARTESIAN_POINT ( 'NONE',  ( 3.775308065498752086, -6.007798216065404873, 24.64249329374151642 ) ) ;
#21894=CARTESIAN_POINT ( 'NONE',  ( -1.614399933863613468, -11.22469193450124969, 22.61124329374151287 ) ) ;
#21980=CARTESIAN_POINT ( 'NONE',  ( 2.651650429449569302, -10.15165042944953733, 25.87500000000000355 ) ) ;
#21988=CARTESIAN_POINT ( 'NONE',  ( 1.614399933863660985, -11.22469193450123193, 16.95125670625848713 ) ) ;
#22003=CARTESIAN_POINT ( 'NONE',  ( 2.724691934501250135, -8.700186371490531201, 21.04874329374151642 ) ) ;
#22108=CARTESIAN_POINT ( 'NONE',  ( 2.608446859217924629, -10.19485399968118422, 13.62686829374151642 ) ) ;
#22116=CARTESIAN_POINT ( 'NONE',  ( -1.139087296526025250, -4.750000000000006217, 15.32812500000000178 ) ) ;
#22213=CARTESIAN_POINT ( 'NONE',  ( 2.750000000000001776, -7.499999999999984013, 23.21875000000000000 ) ) ;
#22281=CARTESIAN_POINT ( 'NONE',  ( 2.320192649118979489E-14, -11.25000000000000000, 24.78125000000000000 ) ) ;
#22312=CARTESIAN_POINT ( 'NONE',  ( 1.901340078031349856, -5.512252781505337929, 24.06063170625849423 ) ) ;
#22315=CARTESIAN_POINT ( 'NONE',  ( -1.196977438190478971, -3.948374222870081773, 14.00000000000000000 ) ) ;
#22324=CARTESIAN_POINT ( 'NONE',  ( 1.901340078031349856, -5.512252781505337929, 25.31063170625848713 ) ) ;
#22332=CARTESIAN_POINT ( 'NONE',  ( -3.749999999999988454, -9.053300858899127945, 18.76562500000000000 ) ) ;
#22337=CARTESIAN_POINT ( 'NONE',  ( 2.651650429449539104, -4.848349570550432475, 18.06250000000000355 ) ) ;
#22416=CARTESIAN_POINT ( 'NONE',  ( -3.749999999999996447, -7.561099074964554134, 22.34188170625849068 ) ) ;
#22426=CARTESIAN_POINT ( 'NONE',  ( -3.775308065498766297, -6.007798216065450170, 19.92000670625849068 ) ) ;
#22441=CARTESIAN_POINT ( 'NONE',  ( 1.901340078031373171, -9.487747218494639867, 19.87686829374151287 ) ) ;
#22476=EDGE_CURVE ( 'NONE', #58074, #28286, #60345, .T. ) ;
#22522=CARTESIAN_POINT ( 'NONE',  ( 2.651650429449539104, -4.848349570550432475, 15.56250000000000000 ) ) ;
#22533=CARTESIAN_POINT ( 'NONE',  ( 3.750000000000000888, -7.499999999999978684, 15.71875000000000000 ) ) ;
#22547=CARTESIAN_POINT ( 'NONE',  ( 2.750000000000002665, -7.561099074964516831, 24.72061829374150932 ) ) ;
#22551=CARTESIAN_POINT ( 'NONE',  ( -1.139087296526025916, -4.750000000000006217, 19.07812500000000000 ) ) ;
#22556=CARTESIAN_POINT ( 'NONE',  ( 1.799775606325937360E-14, -10.25000000000000000, 16.03125000000000000 ) ) ;
#22649=CARTESIAN_POINT ( 'NONE',  ( 1.139087296525997273, -4.749999999999992895, 21.73437500000000000 ) ) ;
#22714=CARTESIAN_POINT ( 'NONE',  ( 2.651650429449539104, -4.848349570550432475, 25.56250000000000355 ) ) ;
#22746=CARTESIAN_POINT ( 'NONE',  ( 1.200186371490561621, -10.22469193450123193, 21.95125670625849068 ) ) ;
#22757=CARTESIAN_POINT ( 'NONE',  ( 2.750000000000001332, -7.438900925035452083, 25.46688170625849423 ) ) ;
#22764=CARTESIAN_POINT ( 'NONE',  ( 3.750000000000000888, -7.499999999999978684, 15.71875000000000000 ) ) ;
#22770=CARTESIAN_POINT ( 'NONE',  ( -2.651650429449535551, -10.15165042944956753, 16.18750000000000000 ) ) ;
#22812=CARTESIAN_POINT ( 'NONE',  ( -1.553300858899125059, -3.750000000000009326, 19.07812500000000000 ) ) ;
#22852=CARTESIAN_POINT ( 'NONE',  ( -0.06109907496455085213, -3.750000000000000888, 18.90438170625848713 ) ) ;
#22860=CARTESIAN_POINT ( 'NONE',  ( 1.614399933863660985, -11.22469193450123193, 19.45125670625849068 ) ) ;
#22876=CARTESIAN_POINT ( 'NONE',  ( -1.077988221561493543, -4.724691934501247914, 24.32999329374151642 ) ) ;
#22961=CARTESIAN_POINT ( 'NONE',  ( -1.553300858899081538, -11.25000000000000711, 14.85937500000000355 ) ) ;
#22970=CARTESIAN_POINT ( 'NONE',  ( 3.750000000000009770, -9.053300858899081760, 19.54687499999999645 ) ) ;
#22985=CARTESIAN_POINT ( 'NONE',  ( 1.987747218494642309, -5.598659921968629050, 23.31436829374150932 ) ) ;
#22989=CARTESIAN_POINT ( 'NONE',  ( 1.139087296525997273, -4.749999999999992895, 24.23437500000000355 ) ) ;
#23096=CARTESIAN_POINT ( 'NONE',  ( -1.139087296526025916, -4.750000000000006217, 25.32812500000000711 ) ) ;
#23101=( BOUNDED_CURVE ( )  B_SPLINE_CURVE ( 2, ( #73250, #19195, #59734, #3889, #45322, #10221, #72795 ),
 .UNSPECIFIED., .F., .F. ) 
 B_SPLINE_CURVE_WITH_KNOTS ( ( 3, 2, 2, 3 ),
 ( 0.000000000000000000, 0.01250000000000000069, 0.02500000000000000139, 0.03447824448891075727 ),
 .UNSPECIFIED. ) 
 CURVE ( )  GEOMETRIC_REPRESENTATION_ITEM ( )  RATIONAL_B_SPLINE_CURVE ( ( 0.5359370743784122038, 0.4951412937321941765, 0.5359370743784122038, 0.4951412937321941765, 0.5359370743784122038, 0.5050032837319460288, 0.5209811780000378478 ) ) 
 REPRESENTATION_ITEM ( '' )  );
#23164=CARTESIAN_POINT ( 'NONE',  ( 3.750000000000000888, -7.499999999999978684, 24.46875000000000000 ) ) ;
#23198=CARTESIAN_POINT ( 'NONE',  ( 2.750000000000001332, -7.438900925035452083, 22.96688170625849068 ) ) ;
#23200=CARTESIAN_POINT ( 'NONE',  ( 3.255975518055617357, -8.015373823202054382, 14.00000000000003553 ) ) ;
#23207=CARTESIAN_POINT ( 'NONE',  ( 2.724691934501235036, -6.299813628509441266, 22.88875670625849068 ) ) ;
#23214=CARTESIAN_POINT ( 'NONE',  ( -3.749999999999997335, -7.500000000000021316, 17.59375000000000000 ) ) ;
#23219=CARTESIAN_POINT ( 'NONE',  ( -3.749999999999997335, -7.500000000000021316, 18.84375000000000000 ) ) ;
#23254=CARTESIAN_POINT ( 'NONE',  ( 1.553300858899087311, -3.749999999999992006, 22.98437500000000000 ) ) ;
#23295=CARTESIAN_POINT ( 'NONE',  ( 1.614399933863660985, -11.22469193450123193, 21.95125670625849068 ) ) ;
#23304=CARTESIAN_POINT ( 'NONE',  ( 2.694853999681214862, -10.10844685921789043, 21.87313170625849068 ) ) ;
#23319=CARTESIAN_POINT ( 'NONE',  ( -2.608446859217920633, -4.805146000318815780, 14.25186829374151465 ) ) ;
#23397=CARTESIAN_POINT ( 'NONE',  ( 3.749999999999992006, -5.946699141100872943, 16.89062500000000000 ) ) ;
#23407=CARTESIAN_POINT ( 'NONE',  ( 1.553300858899087311, -3.749999999999992006, 19.23437500000000355 ) ) ;
#23421=CARTESIAN_POINT ( 'NONE',  ( 2.608446859217924629, -10.19485399968118422, 18.62686829374151642 ) ) ;
#23426=CARTESIAN_POINT ( 'NONE',  ( 2.750000000000008438, -8.639087296525996607, 24.54687500000000000 ) ) ;
#23428=EDGE_CURVE ( 'NONE', #73515, #25338, #612, .T. ) ;
#23433=CARTESIAN_POINT ( 'NONE',  ( -1.944543648262992530, -9.444543648263016067, 19.93750000000000000 ) ) ;
#23527=CARTESIAN_POINT ( 'NONE',  ( 2.750000000000001776, -7.499999999999984013, 24.46875000000000000 ) ) ;
#23610=( BOUNDED_SURFACE ( )  B_SPLINE_SURFACE ( 3, 2, ( 
 ( #25851, #77031, #80810, #12335, #67283, #3569, #30168, #64818, #9451, #79243, #58071, #22961, #29731, #72029, #1805, #84244, #30598, #44102, #49987, #9890, #22522, #17544, #56749, #65271, #2674, #50422, #2236, #77468, #57633, #31038, #15776, #16209, #44545, #36051, #44996, #37351, #43240, #23397, #70716, #86000, #77904, #58503, #50854, #72476, #57193, #24281, #9018, #36487, #43672, #78340, #71144, #85116, #36913, #51740, #63939, #71582, #85555, #64376, #63502, #29293, #16642, #84686, #3124, #23828, #51284, #78788, #17091, #10340, #37805, #39610, #53988, #67513, #4926, #67067, #73376, #81478, #32834, #86918, #4469, #46792, #65712, #58962, #5366, #18875, #24739, #73833, #86465, #19765, #31498, #40053, #66623, #25186, #66162, #52201, #32390, #5808, #79690, #80134, #19323, #10784, #47225, #12129, #17993, #87354, #45445, #60745, #52650, #33285, #25631, #38256, #31951, #88251, #72927, #11230, #18435, #53088, #45893, #59857, #11683, #26527, #4008, #74268, #26078, #38700, #59415, #39161, #80593, #46346, #60298, #87808, #53538, #81035, #12566, #68831, #56207, #62942, #20212, #40924, #13444, #6688, #41817, #13886, #34159, #74719, #89131, #14786, #1253, #67956, #27407, #69719, #83696, #54878, #21980, #75160, #8024, #28743, #13008, #20643, #42261, #82361, #35492 ),
 ( #76029, #83241, #62502, #75582, #40492, #62072, #47675, #41368, #7137, #27848, #48108, #61625, #35044, #55312, #6259, #34608, #68388, #384, #69281, #82805, #21078, #33722, #48547, #61179, #88691, #26971, #14332, #54426, #81920, #7582, #817, #28284, #55754, #21531, #49005, #76482, #16988, #63844, #78694, #85015, #16541, #63397, #50755, #77800, #43570, #3018, #57084, #49883, #71478, #9787, #22852, #35943, #51186, #44438, #2139, #30064, #77362, #36814, #84580, #30931, #70160, #57528, #44008, #50316, #71927, #10241, #64274, #84141, #49452, #70607, #15228, #16105, #58399, #8912, #85897, #78239, #3465, #37698, #71045, #37246, #9357, #76924, #64718, #36382, #43138, #85451, #42700, #8470, #30499, #23295, #1705, #57970, #29195, #56647, #22416, #65164, #2572, #29628, #15668, #23731, #45789, #80929, #38146, #4364, #32719, #24181, #5691, #87246, #3905, #11574, #58856, #74157, #11120, #46679, #39055, #60630, #79588, #53426, #65604, #86361, #66052, #66512, #38596, #18326, #31846, #19214, #12452, #87687, #39498, #51632, #39939, #79137, #59302, #24633, #67398, #72812, #73727, #33167, #17438, #73267, #44892, #72369, #52097, #17885, #25078, #45339, #86808, #66957, #4816, #52541, #10680, #31392, #80024, #32286, #59751, #25526, #18773, #52981, #80477, #46241, #12021 ),
 ( #5252, #60186, #25962, #26414, #34051, #20536, #40818, #82249, #47999, #40381, #55206, #68725, #88584, #67841, #75927, #14673, #82698, #20096, #35380, #61514, #69172, #55643, #81808, #41699, #19650, #6140, #53880, #47111, #81365, #7021, #14226, #68281, #270, #7477, #34930, #89021, #69609, #75478, #33614, #54761, #13776, #41261, #6586, #47560, #48439, #34496, #7915, #27296, #20968, #61959, #61077, #74602, #75051, #88141, #27733, #26855, #54314, #13336, #62394, #83135, #710, #28175, #21426, #48893, #76364, #42154, #12890, #29961, #10128, #9255, #57419, #1601, #49777, #8807, #43911, #64610, #36713, #71373, #9681, #15562, #37147, #2036, #84033, #76821, #70944, #84470, #78581, #2909, #23636, #22746, #42592, #77252, #70052, #15119, #43470, #63291, #43030, #62832, #77694, #56097, #30400, #57868, #23198, #21869, #84914, #51088, #70500, #36280, #85351, #16883, #64168, #44337, #71823, #63734, #1153, #29521, #22312, #8362, #2469, #50208, #28634, #83592, #49345, #16005, #35836, #56976, #29089, #56542, #50659, #78140, #16443, #74065, #52440, #30837, #5153, #32620, #87147, #85800, #32186, #25871, #38497, #31292, #65512, #80383, #59202, #24523, #60088, #87592, #53329, #17787, #80833, #66858, #59646, #19116, #86707, #72269, #24973, #45690, #73171, #46582, #38952 ),
 ( #58759, #4715, #65954, #86255, #37594, #51991, #65057, #3365, #58306, #79486, #24081, #51529, #45239, #79031, #38048, #17331, #44788, #10579, #72714, #3812, #11025, #4261, #11470, #25424, #31743, #66410, #79925, #18229, #18678, #52883, #46143, #73631, #11921, #39398, #88050, #14125, #41601, #54213, #82152, #12797, #88925, #19992, #83033, #33069, #20444, #6920, #13244, #34834, #69071, #27197, #47012, #12359, #33521, #67304, #74955, #21319, #60978, #48791, #41160, #55549, #7378, #6490, #68624, #40725, #39835, #34393, #88482, #26754, #61856, #5599, #60536, #33951, #26313, #615, #74498, #67744, #40283, #81708, #168, #68188, #47458, #53779, #61412, #62301, #28084, #81267, #54654, #19551, #6049, #47906, #75387, #13680, #27638, #55109, #82603, #20876, #48345, #75822, #16340, #22649, #43369, #1056, #77600, #15465, #70406, #29859, #83932, #76717, #9154, #36615, #49680, #62740, #78036, #43804, #28988, #56875, #15019, #63635, #22213, #57765, #7816, #84370, #70852, #77157, #9575, #71266, #1941, #21768, #76261, #8265, #42053, #42936, #85249, #35738, #23527, #15908, #30298, #37038, #8708, #64071, #36186, #14567, #2366, #63188, #69952, #23096, #69509, #35282, #57323, #50115, #28532, #84819, #55994, #83486, #49244, #64498, #29427, #1504, #42493, #56443, #50558 ),
 ( #2806, #24861, #30731, #38385, #85688, #11810, #37941, #73514, #65840, #87483, #17220, #80268, #64953, #23967, #3697, #4141, #65405, #45132, #31171, #18564, #46028, #25317, #66297, #50982, #39289, #78472, #58643, #51416, #66745, #59091, #3258, #52331, #37485, #32509, #71714, #5043, #17676, #86137, #44676, #10018, #72607, #59986, #58197, #24411, #59538, #16773, #44226, #79825, #78920, #31629, #72160, #10474, #51876, #79373, #86590, #10915, #18121, #45580, #73058, #11354, #38838, #4599, #32073, #87042, #52778, #82494, #20774, #65, #41055, #25763, #55006, #53222, #40178, #26204, #14017, #74394, #75285, #68960, #34734, #19887, #7268, #41494, #60429, #81162, #53674, #46908, #82047, #54106, #12693, #80726, #67641, #48239, #62202, #19006, #5942, #75712, #46478, #33412, #73957, #19447, #12247, #39732, #67200, #60874, #5500, #88376, #32964, #61301, #20343, #87944, #27088, #81601, #47354, #68515, #26649, #74849, #47803, #13574, #13138, #40618, #27537, #68087, #6391, #33845, #88817, #54550, #6813, #34287, #61747, #8599, #84268, #1388, #22985, #57221, #15356, #35177, #511, #21662, #55446, #63077, #9473, #49132, #36937, #29317, #43698, #84712, #83825, #56771, #28880, #71168, #22547, #76610, #83374, #36513, #82930, #48682, #50014, #27977, #35631, #50450, #14917 ),
 ( #42395, #1830, #9043, #77489, #56338, #21214, #77056, #62635, #22108, #49578, #42830, #8155, #69852, #15802, #70293, #76156, #36075, #43266, #63526, #41944, #14465, #70741, #69410, #63963, #7718, #948, #2259, #29754, #77929, #16232, #28418, #55886, #12043, #33187, #78813, #57660, #32738, #12913, #39516, #60208, #3148, #51308, #10366, #46699, #67418, #66979, #74176, #12475, #17113, #39959, #3594, #85580, #78366, #73748, #86027, #81388, #5715, #26437, #24305, #44126, #44568, #71606, #16667, #46258, #64846, #72055, #64400, #79270, #85142, #60651, #88162, #25984, #23421, #87712, #53900, #65298, #58096, #30624, #19236, #51766, #37828, #19670, #47133, #74623, #31063, #2699, #30195, #53447, #50879, #17571, #9913, #5274, #80950, #37376, #23855, #58530, #76842, #28193, #61534, #13799, #67860, #75498, #61981, #82270, #34518, #289, #81829, #7497, #20989, #40839, #20122, #55663, #56119, #34953, #89041, #40403, #41282, #21444, #27319, #54334, #48460, #27755, #83610, #48915, #1170, #55227, #47583, #54781, #75071, #13357, #75946, #68302, #20557, #6163, #82716, #33634, #7934, #35400, #729, #88605, #62414, #28652, #68744, #34072, #6605, #83153, #14246, #48020, #62852, #21889, #49364, #7042, #61096, #69629, #76387, #26877, #41725, #69189, #14691, #42176, #50675 ),
 ( #70523, #43048, #36298, #71394, #43490, #63755, #15139, #29539, #44355, #3385, #8381, #56997, #10153, #85818, #84489, #24098, #15581, #1621, #9699, #2058, #77715, #71844, #22764, #37615, #78160, #37169, #29107, #16462, #70963, #9273, #57885, #50227, #8828, #64630, #2933, #16022, #56563, #16904, #65077, #36732, #84935, #64185, #2490, #29979, #51548, #35854, #23214, #30420, #57437, #30854, #58325, #43929, #49797, #42612, #85370, #70074, #23656, #63314, #51106, #84052, #78600, #22332, #77272, #73189, #18696, #52458, #33085, #11940, #65972, #72730, #25887, #44807, #38066, #73648, #87165, #3831, #52900, #65529, #60554, #10599, #39417, #59666, #88067, #31765, #66877, #25444, #31311, #58775, #38515, #79048, #11487, #86275, #24544, #4277, #11042, #74081, #46163, #52011, #4733, #80399, #46604, #59221, #72286, #5171, #26329, #32638, #60109, #17805, #86727, #24992, #87608, #80850, #53351, #19131, #12376, #79944, #39854, #18246, #45708, #79504, #67320, #38972, #5615, #17352, #45258, #66430, #32209, #68206, #60997, #6066, #34409, #54230, #6507, #1072, #68641, #47031, #21339, #48806, #14142, #12812, #48363, #42071, #54671, #47474, #81727, #7395, #75405, #40741, #76279, #14585, #69526, #33966, #7832, #83052, #75841, #35298, #13698, #88499, #41176, #61873, #188 ) ),
 .UNSPECIFIED., .T., .F., .F. ) 
 B_SPLINE_SURFACE_WITH_KNOTS ( ( 4, 3, 4 ),
 ( 3, 2, 2, 2, 2, 2, 2, 2, 2, 2, 2, 2, 2, 2, 2, 2, 2, 2, 2, 2, 2, 2, 2, 2, 2, 2, 2, 2, 2, 2, 2, 2, 2, 2, 2, 2, 2, 2, 2, 2, 2, 2, 2, 2, 2, 2, 2, 2, 2, 2, 2, 2, 2, 2, 2, 2, 2, 2, 2, 2, 2, 2, 2, 2, 2, 2, 2, 2, 2, 2, 2, 2, 2, 2, 2, 2, 2, 2, 2, 2, 3 ),
 ( 0.000000000000000000, 0.5000000000000000000, 1.000000000000000000 ),
 ( 0.000000000000000000, 0.01250000000000000069, 0.02500000000000000139, 0.03749999999999999861, 0.05000000000000000278, 0.06250000000000000000, 0.07499999999999999722, 0.08749999999999999445, 0.1000000000000000056, 0.1125000000000000028, 0.1250000000000000000, 0.1375000000000000111, 0.1499999999999999944, 0.1625000000000000056, 0.1749999999999999889, 0.1875000000000000000, 0.2000000000000000111, 0.2124999999999999944, 0.2250000000000000056, 0.2374999999999999889, 0.2500000000000000000, 0.2625000000000000111, 0.2750000000000000222, 0.2874999999999999778, 0.2999999999999999889, 0.3125000000000000000, 0.3250000000000000111, 0.3375000000000000222, 0.3499999999999999778, 0.3624999999999999889, 0.3750000000000000000, 0.3875000000000000111, 0.4000000000000000222, 0.4124999999999999778, 0.4249999999999999889, 0.4375000000000000000, 0.4500000000000000111, 0.4625000000000000222, 0.4749999999999999778, 0.4874999999999999889, 0.5000000000000000000, 0.5124999999999999556, 0.5250000000000000222, 0.5374999999999999778, 0.5500000000000000444, 0.5625000000000000000, 0.5749999999999999556, 0.5875000000000000222, 0.5999999999999999778, 0.6125000000000000444, 0.6250000000000000000, 0.6374999999999999556, 0.6500000000000000222, 0.6624999999999999778, 0.6750000000000000444, 0.6875000000000000000, 0.6999999999999999556, 0.7125000000000000222, 0.7249999999999999778, 0.7375000000000000444, 0.7500000000000000000, 0.7624999999999999556, 0.7750000000000000222, 0.7874999999999999778, 0.8000000000000000444, 0.8125000000000000000, 0.8249999999999999556, 0.8375000000000000222, 0.8499999999999999778, 0.8625000000000000444, 0.8750000000000000000, 0.8874999999999999556, 0.9000000000000000222, 0.9124999999999999778, 0.9250000000000000444, 0.9375000000000000000, 0.9499999999999999556, 0.9625000000000000222, 0.9749999999999999778, 0.9875000000000000444, 1.000000000000000000 ),
 .UNSPECIFIED. ) 
 GEOMETRIC_REPRESENTATION_ITEM ( )  RATIONAL_B_SPLINE_SURFACE ( (
 ( 1.000000000000000000, 0.9238795325112867385, 1.000000000000000000, 0.9238795325112867385, 1.000000000000000000, 0.9238795325112867385, 1.000000000000000000, 0.9238795325112867385, 1.000000000000000000, 0.9238795325112867385, 1.000000000000000000, 0.9238795325112867385, 1.000000000000000000, 0.9238795325112867385, 1.000000000000000000, 0.9238795325112867385, 1.000000000000000000, 0.9238795325112867385, 1.000000000000000000, 0.9238795325112867385, 1.000000000000000000, 0.9238795325112867385, 1.000000000000000000, 0.9238795325112867385, 1.000000000000000000, 0.9238795325112867385, 1.000000000000000000, 0.9238795325112867385, 1.000000000000000000, 0.9238795325112867385, 1.000000000000000000, 0.9238795325112867385, 1.000000000000000000, 0.9238795325112867385, 1.000000000000000000, 0.9238795325112867385, 1.000000000000000000, 0.9238795325112867385, 1.000000000000000000, 0.9238795325112867385, 1.000000000000000000, 0.9238795325112867385, 1.000000000000000000, 0.9238795325112867385, 1.000000000000000000, 0.9238795325112867385, 1.000000000000000000, 0.9238795325112867385, 1.000000000000000000, 0.9238795325112867385, 1.000000000000000000, 0.9238795325112867385, 1.000000000000000000, 0.9238795325112867385, 1.000000000000000000, 0.9238795325112867385, 1.000000000000000000, 0.9238795325112867385, 1.000000000000000000, 0.9238795325112867385, 1.000000000000000000, 0.9238795325112867385, 1.000000000000000000, 0.9238795325112867385, 1.000000000000000000, 0.9238795325112867385, 1.000000000000000000, 0.9238795325112867385, 1.000000000000000000, 0.9238795325112867385, 1.000000000000000000, 0.9238795325112867385, 1.000000000000000000, 0.9238795325112867385, 1.000000000000000000, 0.9238795325112867385, 1.000000000000000000, 0.9238795325112867385, 1.000000000000000000, 0.9238795325112867385, 1.000000000000000000, 0.9238795325112867385, 1.000000000000000000, 0.9238795325112867385, 1.000000000000000000, 0.9238795325112867385, 1.000000000000000000, 0.9238795325112867385, 1.000000000000000000, 0.9238795325112867385, 1.000000000000000000, 0.9238795325112867385, 1.000000000000000000, 0.9238795325112867385, 1.000000000000000000, 0.9238795325112867385, 1.000000000000000000, 0.9238795325112867385, 1.000000000000000000, 0.9238795325112867385, 1.000000000000000000, 0.9238795325112867385, 1.000000000000000000, 0.9238795325112867385, 1.000000000000000000, 0.9238795325112867385, 1.000000000000000000, 0.9238795325112867385, 1.000000000000000000, 0.9238795325112867385, 1.000000000000000000, 0.9238795325112867385, 1.000000000000000000, 0.9238795325112867385, 1.000000000000000000, 0.9238795325112867385, 1.000000000000000000, 0.9238795325112867385, 1.000000000000000000, 0.9238795325112867385, 1.000000000000000000, 0.9238795325112867385, 1.000000000000000000, 0.9238795325112867385, 1.000000000000000000, 0.9238795325112867385, 1.000000000000000000, 0.9238795325112867385, 1.000000000000000000, 0.9238795325112867385, 1.000000000000000000, 0.9238795325112867385, 1.000000000000000000, 0.9238795325112867385, 1.000000000000000000, 0.9238795325112867385, 1.000000000000000000, 0.9238795325112867385, 1.000000000000000000, 0.9238795325112867385, 1.000000000000000000, 0.9238795325112867385, 1.000000000000000000, 0.9238795325112867385, 1.000000000000000000, 0.9238795325112867385, 1.000000000000000000, 0.9238795325112867385, 1.000000000000000000, 0.9238795325112867385, 1.000000000000000000, 0.9238795325112867385, 1.000000000000000000, 0.9238795325112867385, 1.000000000000000000, 0.9238795325112867385, 1.000000000000000000, 0.9238795325112867385, 1.000000000000000000, 0.9238795325112867385, 1.000000000000000000),
 ( 0.3333333333333333703, 0.3079598441704289313, 0.3333333333333333703, 0.3079598441704289313, 0.3333333333333333703, 0.3079598441704289313, 0.3333333333333333703, 0.3079598441704289313, 0.3333333333333333703, 0.3079598441704289313, 0.3333333333333333703, 0.3079598441704289313, 0.3333333333333333703, 0.3079598441704289313, 0.3333333333333333703, 0.3079598441704289313, 0.3333333333333333703, 0.3079598441704289313, 0.3333333333333333703, 0.3079598441704289313, 0.3333333333333333703, 0.3079598441704289313, 0.3333333333333333703, 0.3079598441704289313, 0.3333333333333333703, 0.3079598441704289313, 0.3333333333333333703, 0.3079598441704289313, 0.3333333333333333703, 0.3079598441704289313, 0.3333333333333333703, 0.3079598441704289313, 0.3333333333333333703, 0.3079598441704289313, 0.3333333333333333703, 0.3079598441704289313, 0.3333333333333333703, 0.3079598441704289313, 0.3333333333333333703, 0.3079598441704289313, 0.3333333333333333703, 0.3079598441704289313, 0.3333333333333333703, 0.3079598441704289313, 0.3333333333333333703, 0.3079598441704289313, 0.3333333333333333703, 0.3079598441704289313, 0.3333333333333333703, 0.3079598441704289313, 0.3333333333333333703, 0.3079598441704289313, 0.3333333333333333703, 0.3079598441704289313, 0.3333333333333333703, 0.3079598441704289313, 0.3333333333333333703, 0.3079598441704289313, 0.3333333333333333703, 0.3079598441704289313, 0.3333333333333333703, 0.3079598441704289313, 0.3333333333333333703, 0.3079598441704289313, 0.3333333333333333703, 0.3079598441704289313, 0.3333333333333333703, 0.3079598441704289313, 0.3333333333333333703, 0.3079598441704289313, 0.3333333333333333703, 0.3079598441704289313, 0.3333333333333333703, 0.3079598441704289313, 0.3333333333333333703, 0.3079598441704289313, 0.3333333333333333703, 0.3079598441704289313, 0.3333333333333333703, 0.3079598441704289313, 0.3333333333333333703, 0.3079598441704289313, 0.3333333333333333703, 0.3079598441704289313, 0.3333333333333333703, 0.3079598441704289313, 0.3333333333333333703, 0.3079598441704289313, 0.3333333333333333703, 0.3079598441704289313, 0.3333333333333333703, 0.3079598441704289313, 0.3333333333333333703, 0.3079598441704289313, 0.3333333333333333703, 0.3079598441704289313, 0.3333333333333333703, 0.3079598441704289313, 0.3333333333333333703, 0.3079598441704289313, 0.3333333333333333703, 0.3079598441704289313, 0.3333333333333333703, 0.3079598441704289313, 0.3333333333333333703, 0.3079598441704289313, 0.3333333333333333703, 0.3079598441704289313, 0.3333333333333333703, 0.3079598441704289313, 0.3333333333333333703, 0.3079598441704289313, 0.3333333333333333703, 0.3079598441704289313, 0.3333333333333333703, 0.3079598441704289313, 0.3333333333333333703, 0.3079598441704289313, 0.3333333333333333703, 0.3079598441704289313, 0.3333333333333333703, 0.3079598441704289313, 0.3333333333333333703, 0.3079598441704289313, 0.3333333333333333703, 0.3079598441704289313, 0.3333333333333333703, 0.3079598441704289313, 0.3333333333333333703, 0.3079598441704289313, 0.3333333333333333703, 0.3079598441704289313, 0.3333333333333333703, 0.3079598441704289313, 0.3333333333333333703, 0.3079598441704289313, 0.3333333333333333703, 0.3079598441704289313, 0.3333333333333333703, 0.3079598441704289313, 0.3333333333333333703, 0.3079598441704289313, 0.3333333333333333703, 0.3079598441704289313, 0.3333333333333333703, 0.3079598441704289313, 0.3333333333333333703, 0.3079598441704289313, 0.3333333333333333703, 0.3079598441704289313, 0.3333333333333333703, 0.3079598441704289313, 0.3333333333333333703, 0.3079598441704289313, 0.3333333333333333703, 0.3079598441704289313, 0.3333333333333333703, 0.3079598441704289313, 0.3333333333333333703, 0.3079598441704289313, 0.3333333333333333703),
 ( 0.3333333333333333703, 0.3079598441704289313, 0.3333333333333333703, 0.3079598441704289313, 0.3333333333333333703, 0.3079598441704289313, 0.3333333333333333703, 0.3079598441704289313, 0.3333333333333333703, 0.3079598441704289313, 0.3333333333333333703, 0.3079598441704289313, 0.3333333333333333703, 0.3079598441704289313, 0.3333333333333333703, 0.3079598441704289313, 0.3333333333333333703, 0.3079598441704289313, 0.3333333333333333703, 0.3079598441704289313, 0.3333333333333333703, 0.3079598441704289313, 0.3333333333333333703, 0.3079598441704289313, 0.3333333333333333703, 0.3079598441704289313, 0.3333333333333333703, 0.3079598441704289313, 0.3333333333333333703, 0.3079598441704289313, 0.3333333333333333703, 0.3079598441704289313, 0.3333333333333333703, 0.3079598441704289313, 0.3333333333333333703, 0.3079598441704289313, 0.3333333333333333703, 0.3079598441704289313, 0.3333333333333333703, 0.3079598441704289313, 0.3333333333333333703, 0.3079598441704289313, 0.3333333333333333703, 0.3079598441704289313, 0.3333333333333333703, 0.3079598441704289313, 0.3333333333333333703, 0.3079598441704289313, 0.3333333333333333703, 0.3079598441704289313, 0.3333333333333333703, 0.3079598441704289313, 0.3333333333333333703, 0.3079598441704289313, 0.3333333333333333703, 0.3079598441704289313, 0.3333333333333333703, 0.3079598441704289313, 0.3333333333333333703, 0.3079598441704289313, 0.3333333333333333703, 0.3079598441704289313, 0.3333333333333333703, 0.3079598441704289313, 0.3333333333333333703, 0.3079598441704289313, 0.3333333333333333703, 0.3079598441704289313, 0.3333333333333333703, 0.3079598441704289313, 0.3333333333333333703, 0.3079598441704289313, 0.3333333333333333703, 0.3079598441704289313, 0.3333333333333333703, 0.3079598441704289313, 0.3333333333333333703, 0.3079598441704289313, 0.3333333333333333703, 0.3079598441704289313, 0.3333333333333333703, 0.3079598441704289313, 0.3333333333333333703, 0.3079598441704289313, 0.3333333333333333703, 0.3079598441704289313, 0.3333333333333333703, 0.3079598441704289313, 0.3333333333333333703, 0.3079598441704289313, 0.3333333333333333703, 0.3079598441704289313, 0.3333333333333333703, 0.3079598441704289313, 0.3333333333333333703, 0.3079598441704289313, 0.3333333333333333703, 0.3079598441704289313, 0.3333333333333333703, 0.3079598441704289313, 0.3333333333333333703, 0.3079598441704289313, 0.3333333333333333703, 0.3079598441704289313, 0.3333333333333333703, 0.3079598441704289313, 0.3333333333333333703, 0.3079598441704289313, 0.3333333333333333703, 0.3079598441704289313, 0.3333333333333333703, 0.3079598441704289313, 0.3333333333333333703, 0.3079598441704289313, 0.3333333333333333703, 0.3079598441704289313, 0.3333333333333333703, 0.3079598441704289313, 0.3333333333333333703, 0.3079598441704289313, 0.3333333333333333703, 0.3079598441704289313, 0.3333333333333333703, 0.3079598441704289313, 0.3333333333333333703, 0.3079598441704289313, 0.3333333333333333703, 0.3079598441704289313, 0.3333333333333333703, 0.3079598441704289313, 0.3333333333333333703, 0.3079598441704289313, 0.3333333333333333703, 0.3079598441704289313, 0.3333333333333333703, 0.3079598441704289313, 0.3333333333333333703, 0.3079598441704289313, 0.3333333333333333703, 0.3079598441704289313, 0.3333333333333333703, 0.3079598441704289313, 0.3333333333333333703, 0.3079598441704289313, 0.3333333333333333703, 0.3079598441704289313, 0.3333333333333333703, 0.3079598441704289313, 0.3333333333333333703, 0.3079598441704289313, 0.3333333333333333703, 0.3079598441704289313, 0.3333333333333333703, 0.3079598441704289313, 0.3333333333333333703, 0.3079598441704289313, 0.3333333333333333703, 0.3079598441704289313, 0.3333333333333333703, 0.3079598441704289313, 0.3333333333333333703),
 ( 1.000000000000000000, 0.9238795325112867385, 1.000000000000000000, 0.9238795325112867385, 1.000000000000000000, 0.9238795325112867385, 1.000000000000000000, 0.9238795325112867385, 1.000000000000000000, 0.9238795325112867385, 1.000000000000000000, 0.9238795325112867385, 1.000000000000000000, 0.9238795325112867385, 1.000000000000000000, 0.9238795325112867385, 1.000000000000000000, 0.9238795325112867385, 1.000000000000000000, 0.9238795325112867385, 1.000000000000000000, 0.9238795325112867385, 1.000000000000000000, 0.9238795325112867385, 1.000000000000000000, 0.9238795325112867385, 1.000000000000000000, 0.9238795325112867385, 1.000000000000000000, 0.9238795325112867385, 1.000000000000000000, 0.9238795325112867385, 1.000000000000000000, 0.9238795325112867385, 1.000000000000000000, 0.9238795325112867385, 1.000000000000000000, 0.9238795325112867385, 1.000000000000000000, 0.9238795325112867385, 1.000000000000000000, 0.9238795325112867385, 1.000000000000000000, 0.9238795325112867385, 1.000000000000000000, 0.9238795325112867385, 1.000000000000000000, 0.9238795325112867385, 1.000000000000000000, 0.9238795325112867385, 1.000000000000000000, 0.9238795325112867385, 1.000000000000000000, 0.9238795325112867385, 1.000000000000000000, 0.9238795325112867385, 1.000000000000000000, 0.9238795325112867385, 1.000000000000000000, 0.9238795325112867385, 1.000000000000000000, 0.9238795325112867385, 1.000000000000000000, 0.9238795325112867385, 1.000000000000000000, 0.9238795325112867385, 1.000000000000000000, 0.9238795325112867385, 1.000000000000000000, 0.9238795325112867385, 1.000000000000000000, 0.9238795325112867385, 1.000000000000000000, 0.9238795325112867385, 1.000000000000000000, 0.9238795325112867385, 1.000000000000000000, 0.9238795325112867385, 1.000000000000000000, 0.9238795325112867385, 1.000000000000000000, 0.9238795325112867385, 1.000000000000000000, 0.9238795325112867385, 1.000000000000000000, 0.9238795325112867385, 1.000000000000000000, 0.9238795325112867385, 1.000000000000000000, 0.9238795325112867385, 1.000000000000000000, 0.9238795325112867385, 1.000000000000000000, 0.9238795325112867385, 1.000000000000000000, 0.9238795325112867385, 1.000000000000000000, 0.9238795325112867385, 1.000000000000000000, 0.9238795325112867385, 1.000000000000000000, 0.9238795325112867385, 1.000000000000000000, 0.9238795325112867385, 1.000000000000000000, 0.9238795325112867385, 1.000000000000000000, 0.9238795325112867385, 1.000000000000000000, 0.9238795325112867385, 1.000000000000000000, 0.9238795325112867385, 1.000000000000000000, 0.9238795325112867385, 1.000000000000000000, 0.9238795325112867385, 1.000000000000000000, 0.9238795325112867385, 1.000000000000000000, 0.9238795325112867385, 1.000000000000000000, 0.9238795325112867385, 1.000000000000000000, 0.9238795325112867385, 1.000000000000000000, 0.9238795325112867385, 1.000000000000000000, 0.9238795325112867385, 1.000000000000000000, 0.9238795325112867385, 1.000000000000000000, 0.9238795325112867385, 1.000000000000000000, 0.9238795325112867385, 1.000000000000000000, 0.9238795325112867385, 1.000000000000000000, 0.9238795325112867385, 1.000000000000000000, 0.9238795325112867385, 1.000000000000000000, 0.9238795325112867385, 1.000000000000000000, 0.9238795325112867385, 1.000000000000000000, 0.9238795325112867385, 1.000000000000000000, 0.9238795325112867385, 1.000000000000000000, 0.9238795325112867385, 1.000000000000000000, 0.9238795325112867385, 1.000000000000000000, 0.9238795325112867385, 1.000000000000000000, 0.9238795325112867385, 1.000000000000000000, 0.9238795325112867385, 1.000000000000000000, 0.9238795325112867385, 1.000000000000000000),
 ( 0.3333333333333333703, 0.3079598441704289313, 0.3333333333333333703, 0.3079598441704289313, 0.3333333333333333703, 0.3079598441704289313, 0.3333333333333333703, 0.3079598441704289313, 0.3333333333333333703, 0.3079598441704289313, 0.3333333333333333703, 0.3079598441704289313, 0.3333333333333333703, 0.3079598441704289313, 0.3333333333333333703, 0.3079598441704289313, 0.3333333333333333703, 0.3079598441704289313, 0.3333333333333333703, 0.3079598441704289313, 0.3333333333333333703, 0.3079598441704289313, 0.3333333333333333703, 0.3079598441704289313, 0.3333333333333333703, 0.3079598441704289313, 0.3333333333333333703, 0.3079598441704289313, 0.3333333333333333703, 0.3079598441704289313, 0.3333333333333333703, 0.3079598441704289313, 0.3333333333333333703, 0.3079598441704289313, 0.3333333333333333703, 0.3079598441704289313, 0.3333333333333333703, 0.3079598441704289313, 0.3333333333333333703, 0.3079598441704289313, 0.3333333333333333703, 0.3079598441704289313, 0.3333333333333333703, 0.3079598441704289313, 0.3333333333333333703, 0.3079598441704289313, 0.3333333333333333703, 0.3079598441704289313, 0.3333333333333333703, 0.3079598441704289313, 0.3333333333333333703, 0.3079598441704289313, 0.3333333333333333703, 0.3079598441704289313, 0.3333333333333333703, 0.3079598441704289313, 0.3333333333333333703, 0.3079598441704289313, 0.3333333333333333703, 0.3079598441704289313, 0.3333333333333333703, 0.3079598441704289313, 0.3333333333333333703, 0.3079598441704289313, 0.3333333333333333703, 0.3079598441704289313, 0.3333333333333333703, 0.3079598441704289313, 0.3333333333333333703, 0.3079598441704289313, 0.3333333333333333703, 0.3079598441704289313, 0.3333333333333333703, 0.3079598441704289313, 0.3333333333333333703, 0.3079598441704289313, 0.3333333333333333703, 0.3079598441704289313, 0.3333333333333333703, 0.3079598441704289313, 0.3333333333333333703, 0.3079598441704289313, 0.3333333333333333703, 0.3079598441704289313, 0.3333333333333333703, 0.3079598441704289313, 0.3333333333333333703, 0.3079598441704289313, 0.3333333333333333703, 0.3079598441704289313, 0.3333333333333333703, 0.3079598441704289313, 0.3333333333333333703, 0.3079598441704289313, 0.3333333333333333703, 0.3079598441704289313, 0.3333333333333333703, 0.3079598441704289313, 0.3333333333333333703, 0.3079598441704289313, 0.3333333333333333703, 0.3079598441704289313, 0.3333333333333333703, 0.3079598441704289313, 0.3333333333333333703, 0.3079598441704289313, 0.3333333333333333703, 0.3079598441704289313, 0.3333333333333333703, 0.3079598441704289313, 0.3333333333333333703, 0.3079598441704289313, 0.3333333333333333703, 0.3079598441704289313, 0.3333333333333333703, 0.3079598441704289313, 0.3333333333333333703, 0.3079598441704289313, 0.3333333333333333703, 0.3079598441704289313, 0.3333333333333333703, 0.3079598441704289313, 0.3333333333333333703, 0.3079598441704289313, 0.3333333333333333703, 0.3079598441704289313, 0.3333333333333333703, 0.3079598441704289313, 0.3333333333333333703, 0.3079598441704289313, 0.3333333333333333703, 0.3079598441704289313, 0.3333333333333333703, 0.3079598441704289313, 0.3333333333333333703, 0.3079598441704289313, 0.3333333333333333703, 0.3079598441704289313, 0.3333333333333333703, 0.3079598441704289313, 0.3333333333333333703, 0.3079598441704289313, 0.3333333333333333703, 0.3079598441704289313, 0.3333333333333333703, 0.3079598441704289313, 0.3333333333333333703, 0.3079598441704289313, 0.3333333333333333703, 0.3079598441704289313, 0.3333333333333333703, 0.3079598441704289313, 0.3333333333333333703, 0.3079598441704289313, 0.3333333333333333703, 0.3079598441704289313, 0.3333333333333333703, 0.3079598441704289313, 0.3333333333333333703, 0.3079598441704289313, 0.3333333333333333703),
 ( 0.3333333333333333703, 0.3079598441704289313, 0.3333333333333333703, 0.3079598441704289313, 0.3333333333333333703, 0.3079598441704289313, 0.3333333333333333703, 0.3079598441704289313, 0.3333333333333333703, 0.3079598441704289313, 0.3333333333333333703, 0.3079598441704289313, 0.3333333333333333703, 0.3079598441704289313, 0.3333333333333333703, 0.3079598441704289313, 0.3333333333333333703, 0.3079598441704289313, 0.3333333333333333703, 0.3079598441704289313, 0.3333333333333333703, 0.3079598441704289313, 0.3333333333333333703, 0.3079598441704289313, 0.3333333333333333703, 0.3079598441704289313, 0.3333333333333333703, 0.3079598441704289313, 0.3333333333333333703, 0.3079598441704289313, 0.3333333333333333703, 0.3079598441704289313, 0.3333333333333333703, 0.3079598441704289313, 0.3333333333333333703, 0.3079598441704289313, 0.3333333333333333703, 0.3079598441704289313, 0.3333333333333333703, 0.3079598441704289313, 0.3333333333333333703, 0.3079598441704289313, 0.3333333333333333703, 0.3079598441704289313, 0.3333333333333333703, 0.3079598441704289313, 0.3333333333333333703, 0.3079598441704289313, 0.3333333333333333703, 0.3079598441704289313, 0.3333333333333333703, 0.3079598441704289313, 0.3333333333333333703, 0.3079598441704289313, 0.3333333333333333703, 0.3079598441704289313, 0.3333333333333333703, 0.3079598441704289313, 0.3333333333333333703, 0.3079598441704289313, 0.3333333333333333703, 0.3079598441704289313, 0.3333333333333333703, 0.3079598441704289313, 0.3333333333333333703, 0.3079598441704289313, 0.3333333333333333703, 0.3079598441704289313, 0.3333333333333333703, 0.3079598441704289313, 0.3333333333333333703, 0.3079598441704289313, 0.3333333333333333703, 0.3079598441704289313, 0.3333333333333333703, 0.3079598441704289313, 0.3333333333333333703, 0.3079598441704289313, 0.3333333333333333703, 0.3079598441704289313, 0.3333333333333333703, 0.3079598441704289313, 0.3333333333333333703, 0.3079598441704289313, 0.3333333333333333703, 0.3079598441704289313, 0.3333333333333333703, 0.3079598441704289313, 0.3333333333333333703, 0.3079598441704289313, 0.3333333333333333703, 0.3079598441704289313, 0.3333333333333333703, 0.3079598441704289313, 0.3333333333333333703, 0.3079598441704289313, 0.3333333333333333703, 0.3079598441704289313, 0.3333333333333333703, 0.3079598441704289313, 0.3333333333333333703, 0.3079598441704289313, 0.3333333333333333703, 0.3079598441704289313, 0.3333333333333333703, 0.3079598441704289313, 0.3333333333333333703, 0.3079598441704289313, 0.3333333333333333703, 0.3079598441704289313, 0.3333333333333333703, 0.3079598441704289313, 0.3333333333333333703, 0.3079598441704289313, 0.3333333333333333703, 0.3079598441704289313, 0.3333333333333333703, 0.3079598441704289313, 0.3333333333333333703, 0.3079598441704289313, 0.3333333333333333703, 0.3079598441704289313, 0.3333333333333333703, 0.3079598441704289313, 0.3333333333333333703, 0.3079598441704289313, 0.3333333333333333703, 0.3079598441704289313, 0.3333333333333333703, 0.3079598441704289313, 0.3333333333333333703, 0.3079598441704289313, 0.3333333333333333703, 0.3079598441704289313, 0.3333333333333333703, 0.3079598441704289313, 0.3333333333333333703, 0.3079598441704289313, 0.3333333333333333703, 0.3079598441704289313, 0.3333333333333333703, 0.3079598441704289313, 0.3333333333333333703, 0.3079598441704289313, 0.3333333333333333703, 0.3079598441704289313, 0.3333333333333333703, 0.3079598441704289313, 0.3333333333333333703, 0.3079598441704289313, 0.3333333333333333703, 0.3079598441704289313, 0.3333333333333333703, 0.3079598441704289313, 0.3333333333333333703, 0.3079598441704289313, 0.3333333333333333703, 0.3079598441704289313, 0.3333333333333333703, 0.3079598441704289313, 0.3333333333333333703),
 ( 1.000000000000000000, 0.9238795325112867385, 1.000000000000000000, 0.9238795325112867385, 1.000000000000000000, 0.9238795325112867385, 1.000000000000000000, 0.9238795325112867385, 1.000000000000000000, 0.9238795325112867385, 1.000000000000000000, 0.9238795325112867385, 1.000000000000000000, 0.9238795325112867385, 1.000000000000000000, 0.9238795325112867385, 1.000000000000000000, 0.9238795325112867385, 1.000000000000000000, 0.9238795325112867385, 1.000000000000000000, 0.9238795325112867385, 1.000000000000000000, 0.9238795325112867385, 1.000000000000000000, 0.9238795325112867385, 1.000000000000000000, 0.9238795325112867385, 1.000000000000000000, 0.9238795325112867385, 1.000000000000000000, 0.9238795325112867385, 1.000000000000000000, 0.9238795325112867385, 1.000000000000000000, 0.9238795325112867385, 1.000000000000000000, 0.9238795325112867385, 1.000000000000000000, 0.9238795325112867385, 1.000000000000000000, 0.9238795325112867385, 1.000000000000000000, 0.9238795325112867385, 1.000000000000000000, 0.9238795325112867385, 1.000000000000000000, 0.9238795325112867385, 1.000000000000000000, 0.9238795325112867385, 1.000000000000000000, 0.9238795325112867385, 1.000000000000000000, 0.9238795325112867385, 1.000000000000000000, 0.9238795325112867385, 1.000000000000000000, 0.9238795325112867385, 1.000000000000000000, 0.9238795325112867385, 1.000000000000000000, 0.9238795325112867385, 1.000000000000000000, 0.9238795325112867385, 1.000000000000000000, 0.9238795325112867385, 1.000000000000000000, 0.9238795325112867385, 1.000000000000000000, 0.9238795325112867385, 1.000000000000000000, 0.9238795325112867385, 1.000000000000000000, 0.9238795325112867385, 1.000000000000000000, 0.9238795325112867385, 1.000000000000000000, 0.9238795325112867385, 1.000000000000000000, 0.9238795325112867385, 1.000000000000000000, 0.9238795325112867385, 1.000000000000000000, 0.9238795325112867385, 1.000000000000000000, 0.9238795325112867385, 1.000000000000000000, 0.9238795325112867385, 1.000000000000000000, 0.9238795325112867385, 1.000000000000000000, 0.9238795325112867385, 1.000000000000000000, 0.9238795325112867385, 1.000000000000000000, 0.9238795325112867385, 1.000000000000000000, 0.9238795325112867385, 1.000000000000000000, 0.9238795325112867385, 1.000000000000000000, 0.9238795325112867385, 1.000000000000000000, 0.9238795325112867385, 1.000000000000000000, 0.9238795325112867385, 1.000000000000000000, 0.9238795325112867385, 1.000000000000000000, 0.9238795325112867385, 1.000000000000000000, 0.9238795325112867385, 1.000000000000000000, 0.9238795325112867385, 1.000000000000000000, 0.9238795325112867385, 1.000000000000000000, 0.9238795325112867385, 1.000000000000000000, 0.9238795325112867385, 1.000000000000000000, 0.9238795325112867385, 1.000000000000000000, 0.9238795325112867385, 1.000000000000000000, 0.9238795325112867385, 1.000000000000000000, 0.9238795325112867385, 1.000000000000000000, 0.9238795325112867385, 1.000000000000000000, 0.9238795325112867385, 1.000000000000000000, 0.9238795325112867385, 1.000000000000000000, 0.9238795325112867385, 1.000000000000000000, 0.9238795325112867385, 1.000000000000000000, 0.9238795325112867385, 1.000000000000000000, 0.9238795325112867385, 1.000000000000000000, 0.9238795325112867385, 1.000000000000000000, 0.9238795325112867385, 1.000000000000000000, 0.9238795325112867385, 1.000000000000000000, 0.9238795325112867385, 1.000000000000000000, 0.9238795325112867385, 1.000000000000000000, 0.9238795325112867385, 1.000000000000000000, 0.9238795325112867385, 1.000000000000000000, 0.9238795325112867385, 1.000000000000000000, 0.9238795325112867385, 1.000000000000000000) ) ) 
 REPRESENTATION_ITEM ( '' )  SURFACE ( )  );
#23636=CARTESIAN_POINT ( 'NONE',  ( 1.987747218494664292, -9.401340078031346081, 21.87313170625849068 ) ) ;
#23646=CARTESIAN_POINT ( 'NONE',  ( -2.775308065498764964, -6.422011778438537988, 22.42000670625849068 ) ) ;
#23656=CARTESIAN_POINT ( 'NONE',  ( 2.651650429449569302, -10.15165042944953733, 18.37500000000000355 ) ) ;
#23661=CARTESIAN_POINT ( 'NONE',  ( -1.553300858899125059, -3.750000000000009326, 17.82812500000000000 ) ) ;
#23694=CARTESIAN_POINT ( 'NONE',  ( -1.929879867024197893E-14, -3.750000000000000000, 19.15625000000000000 ) ) ;
#23731=CARTESIAN_POINT ( 'NONE',  ( 1.492201783934554493, -3.724691934501233703, 22.73250670625849068 ) ) ;
#23742=CARTESIAN_POINT ( 'NONE',  ( -1.614399933863656544, -3.775308065498769405, 21.32625670625849423 ) ) ;
#23755=CARTESIAN_POINT ( 'NONE',  ( -0.06109907496450878162, -11.25000000000000000, 16.28311829374151287 ) ) ;
#23828=CARTESIAN_POINT ( 'NONE',  ( -3.750000000000008438, -5.946699141100917352, 18.92187500000000355 ) ) ;
#23839=CARTESIAN_POINT ( 'NONE',  ( 3.749999999999992006, -5.946699141100872943, 16.89062500000000000 ) ) ;
#23855=CARTESIAN_POINT ( 'NONE',  ( -3.749999999999997780, -7.438900925035489387, 20.34561829374151287 ) ) ;
#23860=CARTESIAN_POINT ( 'NONE',  ( -1.200186371490524317, -10.22469193450124791, 13.86124329374151820 ) ) ;
#23865=CARTESIAN_POINT ( 'NONE',  ( 1.139087296525997051, -4.749999999999992895, 17.98437500000000000 ) ) ;
#23894=DIRECTION ( 'NONE',  ( -0.7071067811865510144, 0.7071067811865440200, 0.000000000000000000 ) ) ;
#23967=CARTESIAN_POINT ( 'NONE',  ( -2.775308065498752086, -8.577988221561495763, 14.01749329374151642 ) ) ;
#23995=FILL_AREA_STYLE ('',( #85716 ) ) ;
#24081=CARTESIAN_POINT ( 'NONE',  ( 1.799775606325937360E-14, -10.25000000000000000, 14.78125000000000178 ) ) ;
#24090=CARTESIAN_POINT ( 'NONE',  ( 2.724691934501235036, -6.299813628509441266, 26.63875670625848713 ) ) ;
#24098=CARTESIAN_POINT ( 'NONE',  ( -3.750000000000008438, -5.946699141100917352, 15.17187500000000000 ) ) ;
#24140=CARTESIAN_POINT ( 'NONE',  ( -2.651650429449565305, -4.848349570550461785, 24.00000000000000000 ) ) ;
#24147=CARTESIAN_POINT ( 'NONE',  ( -1.929879867024197893E-14, -3.750000000000000000, 16.65625000000000000 ) ) ;
#24181=CARTESIAN_POINT ( 'NONE',  ( 1.614399933863660985, -11.22469193450123193, 23.20125670625849068 ) ) ;
#24191=CARTESIAN_POINT ( 'NONE',  ( -3.724691934501229262, -9.114399933863657211, 21.01375670625849068 ) ) ;
#24203=CARTESIAN_POINT ( 'NONE',  ( 0.06109907496451268821, -3.749999999999999556, 13.15811829374151642 ) ) ;
#24281=CARTESIAN_POINT ( 'NONE',  ( -3.749999999999988454, -9.053300858899127945, 17.51562500000000000 ) ) ;
#24291=CARTESIAN_POINT ( 'NONE',  ( 1.553300858899129944, -11.24999999999998934, 18.45312500000000355 ) ) ;
#24305=CARTESIAN_POINT ( 'NONE',  ( -0.06109907496450878162, -11.25000000000000000, 17.53311829374151287 ) ) ;
#24311=CARTESIAN_POINT ( 'NONE',  ( -1.944543648263014957, -5.555456351737005249, 26.50000000000000355 ) ) ;
#24316=CARTESIAN_POINT ( 'NONE',  ( -1.944543648263014957, -5.555456351737005249, 20.25000000000000000 ) ) ;
#24411=CARTESIAN_POINT ( 'NONE',  ( -1.200186371490524317, -10.22469193450124791, 16.36124329374151642 ) ) ;
#24523=CARTESIAN_POINT ( 'NONE',  ( -1.200186371490556958, -4.775308065498765409, 26.32625670625849068 ) ) ;
#24534=CARTESIAN_POINT ( 'NONE',  ( -1.987747218494660295, -5.598659921968651254, 26.24813170625849068 ) ) ;
#24544=CARTESIAN_POINT ( 'NONE',  ( -2.651650429449535551, -10.15165042944956753, 21.18750000000000000 ) ) ;
#24591=CARTESIAN_POINT ( 'NONE',  ( 1.553300858899087311, -3.749999999999992006, 20.48437500000000000 ) ) ;
#24633=CARTESIAN_POINT ( 'NONE',  ( 3.724691934501232815, -5.885600066136343678, 25.38875670625849423 ) ) ;
#24642=CARTESIAN_POINT ( 'NONE',  ( -3.749999999999996447, -7.561099074964554134, 27.34188170625848713 ) ) ;
#24655=CARTESIAN_POINT ( 'NONE',  ( -0.06109907496450878162, -11.25000000000000000, 15.03311829374151287 ) ) ;
#24739=CARTESIAN_POINT ( 'NONE',  ( 2.651650429449539104, -4.848349570550432475, 20.56250000000000000 ) ) ;
#24747=CARTESIAN_POINT ( 'NONE',  ( 1.553300858899087311, -3.749999999999992006, 20.48437500000000000 ) ) ;
#24766=CARTESIAN_POINT ( 'NONE',  ( 2.750000000000008438, -8.639087296525996607, 25.79687500000000355 ) ) ;
#24771=CARTESIAN_POINT ( 'NONE',  ( 1.139087296526029469, -10.24999999999999289, 20.95312500000000000 ) ) ;
#24861=CARTESIAN_POINT ( 'NONE',  ( -1.077988221561493543, -4.724691934501247914, 13.07999329374151642 ) ) ;
#24973=CARTESIAN_POINT ( 'NONE',  ( -1.901340078031346525, -9.487747218494661183, 27.18563170625849068 ) ) ;
#24983=CARTESIAN_POINT ( 'NONE',  ( -2.775308065498764964, -6.422011778438537988, 27.42000670625849068 ) ) ;
#24992=CARTESIAN_POINT ( 'NONE',  ( -3.749999999999988454, -9.053300858899127945, 22.51562500000000000 ) ) ;
#25038=CARTESIAN_POINT ( 'NONE',  ( -3.749999999999988454, -9.053300858899127945, 26.26562500000000000 ) ) ;
#25045=CARTESIAN_POINT ( 'NONE',  ( -2.651650429449535551, -10.15165042944956753, 14.93750000000000000 ) ) ;
#25078=CARTESIAN_POINT ( 'NONE',  ( -2.694853999681210865, -4.891553140782108677, 26.24813170625849068 ) ) ;
#25087=CARTESIAN_POINT ( 'NONE',  ( 1.901340078031349856, -5.512252781505337929, 15.31063170625849068 ) ) ;
#25101=CARTESIAN_POINT ( 'NONE',  ( 1.614399933863618797, -3.775308065498751198, 19.48624329374152353 ) ) ;
#25186=CARTESIAN_POINT ( 'NONE',  ( -1.553300858899081538, -11.25000000000000711, 21.10937500000000711 ) ) ;
#25194=CARTESIAN_POINT ( 'NONE',  ( -2.651650429449535551, -10.15165042944956753, 22.43750000000000000 ) ) ;
#25215=CARTESIAN_POINT ( 'NONE',  ( -1.077988221561493543, -4.724691934501247914, 18.07999329374151287 ) ) ;
#25220=CARTESIAN_POINT ( 'NONE',  ( -1.944543648263014957, -5.555456351737005249, 16.50000000000000000 ) ) ;
#25273=CARTESIAN_POINT ( 'NONE',  ( -2.651650429449565305, -4.848349570550461785, 14.00000000000000178 ) ) ;
#25317=CARTESIAN_POINT ( 'NONE',  ( 2.775308065498755195, -6.422011778438505125, 14.64249329374151110 ) ) ;
#25338=VERTEX_POINT ( 'NONE', #25273 ) ;
#25340=( NAMED_UNIT ( * ) PLANE_ANGLE_UNIT ( ) SI_UNIT ( $, .RADIAN. ) );
#25424=CARTESIAN_POINT ( 'NONE',  ( 2.750000000000008438, -8.639087296525996607, 15.79687500000000178 ) ) ;
#25434=CARTESIAN_POINT ( 'NONE',  ( 1.944543648262996083, -5.555456351736983045, 14.31250000000000000 ) ) ;
#25444=CARTESIAN_POINT ( 'NONE',  ( 3.749999999999992006, -5.946699141100872943, 20.64062500000000000 ) ) ;
#25488=CARTESIAN_POINT ( 'NONE',  ( -1.553300858899081538, -11.25000000000000711, 26.10937500000001066 ) ) ;
#25493=CARTESIAN_POINT ( 'NONE',  ( 2.651650429449569302, -10.15165042944953733, 15.87500000000000000 ) ) ;
#25526=CARTESIAN_POINT ( 'NONE',  ( -1.492201783934549164, -11.27530806549876807, 27.10750670625849423 ) ) ;
#25537=CARTESIAN_POINT ( 'NONE',  ( -1.492201783934549164, -11.27530806549876807, 27.10750670625849423 ) ) ;
#25550=CARTESIAN_POINT ( 'NONE',  ( 3.750000000000001776, -7.561099074964511502, 17.22061829374151287 ) ) ;
#25631=CARTESIAN_POINT ( 'NONE',  ( -2.651650429449535551, -10.15165042944956753, 22.43750000000000000 ) ) ;
#25642=CARTESIAN_POINT ( 'NONE',  ( -3.750000000000008438, -5.946699141100917352, 21.42187500000000000 ) ) ;
#25661=CARTESIAN_POINT ( 'NONE',  ( 1.200186371490529202, -4.775308065498752974, 14.48624329374151465 ) ) ;
#25667=CARTESIAN_POINT ( 'NONE',  ( 1.139087296526029469, -10.24999999999999289, 24.70312500000000000 ) ) ;
#25763=CARTESIAN_POINT ( 'NONE',  ( 2.775308065498755195, -6.422011778438505125, 18.39249329374151642 ) ) ;
#25788=( LENGTH_UNIT ( ) NAMED_UNIT ( * ) SI_UNIT ( .MILLI., .METRE. ) );
#25851=CARTESIAN_POINT ( 'NONE',  ( -2.651650429449565305, -4.848349570550461785, 14.00000000000000000 ) ) ;
#25871=CARTESIAN_POINT ( 'NONE',  ( -1.077988221561460236, -10.27530806549876452, 25.85750670625849068 ) ) ;
#25879=CARTESIAN_POINT ( 'NONE',  ( 1.944543648262996083, -5.555456351736983045, 15.56250000000000000 ) ) ;
#25887=CARTESIAN_POINT ( 'NONE',  ( 3.750000000000000888, -7.499999999999978684, 19.46875000000000000 ) ) ;
#25932=CARTESIAN_POINT ( 'NONE',  ( 3.750000000000000888, -7.499999999999978684, 14.46875000000000000 ) ) ;
#25962=CARTESIAN_POINT ( 'NONE',  ( -0.06109907496454585613, -4.750000000000000000, 15.15438170625848890 ) ) ;
#25975=CARTESIAN_POINT ( 'NONE',  ( -0.06109907496455085213, -3.750000000000000888, 26.40438170625848713 ) ) ;
#25984=CARTESIAN_POINT ( 'NONE',  ( 3.724691934501251023, -9.114399933863618131, 18.54874329374151642 ) ) ;
#25991=CARTESIAN_POINT ( 'NONE',  ( 0.06109907496451268821, -3.749999999999999556, 16.90811829374151287 ) ) ;
#26078=CARTESIAN_POINT ( 'NONE',  ( 2.320192649118979489E-14, -11.25000000000000000, 23.53125000000000000 ) ) ;
#26086=CARTESIAN_POINT ( 'NONE',  ( -3.750000000000008438, -5.946699141100917352, 22.67187500000000355 ) ) ;
#26103=CARTESIAN_POINT ( 'NONE',  ( -1.200186371490524317, -10.22469193450124791, 18.86124329374151287 ) ) ;
#26109=CARTESIAN_POINT ( 'NONE',  ( -2.749999999999998224, -7.500000000000015987, 22.59375000000000355 ) ) ;
#26204=CARTESIAN_POINT ( 'NONE',  ( 1.077988221561497539, -10.27530806549875386, 18.70499329374151287 ) ) ;
#26313=CARTESIAN_POINT ( 'NONE',  ( 1.944543648263018731, -9.444543648262994751, 19.62500000000000000 ) ) ;
#26321=CARTESIAN_POINT ( 'NONE',  ( -2.749999999999998224, -7.500000000000015987, 17.59375000000000000 ) ) ;
#26329=CARTESIAN_POINT ( 'NONE',  ( 2.651650429449569302, -10.15165042944953733, 22.12500000000000000 ) ) ;
#26383=CARTESIAN_POINT ( 'NONE',  ( 2.320192649118979489E-14, -11.25000000000000000, 22.28125000000000355 ) ) ;
#26414=CARTESIAN_POINT ( 'NONE',  ( 1.077988221561464899, -4.724691934501233703, 15.23250670625848713 ) ) ;
#26428=CARTESIAN_POINT ( 'NONE',  ( 3.775308065498768517, -8.992201783934554271, 26.79500670625849423 ) ) ;
#26437=CARTESIAN_POINT ( 'NONE',  ( 1.492201783934598236, -11.27530806549875031, 17.45499329374151642 ) ) ;
#26444=CARTESIAN_POINT ( 'NONE',  ( 3.750000000000001776, -7.561099074964511502, 20.97061829374151642 ) ) ;
#26481=DIRECTION ( 'NONE',  ( -0.000000000000000000, -0.000000000000000000, 1.000000000000000000 ) ) ;
#26527=CARTESIAN_POINT ( 'NONE',  ( 3.750000000000009770, -9.053300858899081760, 23.29687500000000000 ) ) ;
#26537=CARTESIAN_POINT ( 'NONE',  ( -3.750000000000008438, -5.946699141100917352, 25.17187500000000000 ) ) ;
#26552=CARTESIAN_POINT ( 'NONE',  ( -1.987747218494638313, -9.401340078031370950, 15.18936829374151465 ) ) ;
#26560=CARTESIAN_POINT ( 'NONE',  ( 1.944543648262996083, -5.555456351736983045, 23.06250000000000000 ) ) ;
#26649=CARTESIAN_POINT ( 'NONE',  ( 0.06109907496451789238, -4.749999999999998224, 21.90811829374151642 ) ) ;
#26731=FACE_OUTER_BOUND ( 'NONE', #68018, .T. ) ;
#26754=CARTESIAN_POINT ( 'NONE',  ( 1.139087296525997273, -4.749999999999992895, 19.23437500000000355 ) ) ;
#26755=EDGE_LOOP ( 'NONE', ( #88368, #53437, #9419, #62148 ) ) ;
#26764=CARTESIAN_POINT ( 'NONE',  ( -1.944543648262992530, -9.444543648263016067, 21.18750000000000000 ) ) ;
#26811=APPLICATION_CONTEXT ( 'automotive_design' ) ;
#26828=CARTESIAN_POINT ( 'NONE',  ( -3.750000000000007550, -5.946699141100917352, 20.17187500000000000 ) ) ;
#26855=CARTESIAN_POINT ( 'NONE',  ( 2.775308065498768517, -8.577988221561467341, 19.29500670625849068 ) ) ;
#26869=CARTESIAN_POINT ( 'NONE',  ( 1.901340078031349856, -5.512252781505337929, 16.56063170625848713 ) ) ;
#26877=CARTESIAN_POINT ( 'NONE',  ( -1.614399933863613468, -11.22469193450124969, 25.11124329374151642 ) ) ;
#26883=CARTESIAN_POINT ( 'NONE',  ( -2.608446859217920633, -4.805146000318815780, 24.25186829374150932 ) ) ;
#26971=CARTESIAN_POINT ( 'NONE',  ( 1.614399933863660985, -11.22469193450123193, 16.95125670625848713 ) ) ;
#26980=CARTESIAN_POINT ( 'NONE',  ( -3.775308065498766297, -6.007798216065450170, 17.42000670625848713 ) ) ;
#26993=CARTESIAN_POINT ( 'NONE',  ( 1.987747218494642309, -5.598659921968629050, 14.56436829374151287 ) ) ;
#26999=CARTESIAN_POINT ( 'NONE',  ( -1.409462824231155764E-14, -4.749999999999999112, 25.40625000000000000 ) ) ;
#27088=CARTESIAN_POINT ( 'NONE',  ( -2.749999999999999112, -7.438900925035484057, 21.59561829374151287 ) ) ;
#27197=CARTESIAN_POINT ( 'NONE',  ( -1.139087296526025916, -4.750000000000006217, 17.82812500000000000 ) ) ;
#27206=CARTESIAN_POINT ( 'NONE',  ( -2.750000000000007105, -6.360912703474006946, 20.17187500000000000 ) ) ;
#27263=CARTESIAN_POINT ( 'NONE',  ( -3.749999999999988454, -9.053300858899127945, 22.51562500000000000 ) ) ;
#27296=CARTESIAN_POINT ( 'NONE',  ( -2.775308065498764964, -6.422011778438537988, 18.67000670625849068 ) ) ;
#27309=CARTESIAN_POINT ( 'NONE',  ( 1.987747218494664292, -9.401340078031346081, 18.12313170625849068 ) ) ;
#27318=STYLED_ITEM ( 'NONE', ( #72632 ), #37432 ) ;
#27319=CARTESIAN_POINT ( 'NONE',  ( 3.750000000000001776, -7.561099074964511502, 22.22061829374151287 ) ) ;
#27325=CARTESIAN_POINT ( 'NONE',  ( -1.553300858899125059, -3.750000000000009326, 14.07812500000000178 ) ) ;
#27407=CARTESIAN_POINT ( 'NONE',  ( 2.651650429449539104, -4.848349570550432475, 25.56250000000000355 ) ) ;
#27416=CARTESIAN_POINT ( 'NONE',  ( 2.694853999681214862, -10.10844685921789043, 15.62313170625848890 ) ) ;
#27434=CARTESIAN_POINT ( 'NONE',  ( 0.06109907496451789238, -4.749999999999998224, 21.90811829374151642 ) ) ;
#27441=CARTESIAN_POINT ( 'NONE',  ( 2.750000000000001776, -7.499999999999984013, 25.71875000000000000 ) ) ;
#27537=CARTESIAN_POINT ( 'NONE',  ( 1.901340078031373171, -9.487747218494639867, 22.37686829374150932 ) ) ;
#27543=( NAMED_UNIT ( * ) SI_UNIT ( $, .STERADIAN. ) SOLID_ANGLE_UNIT ( ) );
#27588=CARTESIAN_POINT ( 'NONE',  ( -1.553300858899125059, -3.750000000000009326, 24.07812500000000355 ) ) ;
#27638=CARTESIAN_POINT ( 'NONE',  ( -1.944543648262992530, -9.444543648263016067, 21.18750000000000000 ) ) ;
#27646=CARTESIAN_POINT ( 'NONE',  ( 2.749999999999995115, -6.360912703473971419, 19.39062500000000711 ) ) ;
#27704=CARTESIAN_POINT ( 'NONE',  ( -1.929879867024197893E-14, -3.750000000000000000, 19.15625000000000000 ) ) ;
#27733=CARTESIAN_POINT ( 'NONE',  ( 2.750000000000001332, -7.438900925035452083, 19.21688170625848358 ) ) ;
#27748=CARTESIAN_POINT ( 'NONE',  ( -2.724691934501232371, -8.700186371490559623, 19.76375670625849423 ) ) ;
#27755=CARTESIAN_POINT ( 'NONE',  ( 1.492201783934598236, -11.27530806549875031, 22.45499329374151287 ) ) ;
#27761=CARTESIAN_POINT ( 'NONE',  ( 3.750000000000000888, -7.499999999999978684, 14.46875000000000000 ) ) ;
#27803=DIRECTION ( 'NONE',  ( 1.000000000000000000, 0.000000000000000000, 0.000000000000000000 ) ) ;
#27848=CARTESIAN_POINT ( 'NONE',  ( 1.614399933863660985, -11.22469193450123193, 15.70125670625848890 ) ) ;
#27856=CARTESIAN_POINT ( 'NONE',  ( 3.749999999999992006, -5.946699141100872943, 25.64062500000000000 ) ) ;
#27871=CARTESIAN_POINT ( 'NONE',  ( -1.200186371490524317, -10.22469193450124791, 23.86124329374151998 ) ) ;
#27977=CARTESIAN_POINT ( 'NONE',  ( -2.775308065498752086, -8.577988221561495763, 25.26749329374151642 ) ) ;
#28084=CARTESIAN_POINT ( 'NONE',  ( 1.944543648262996083, -5.555456351736983045, 20.56250000000000000 ) ) ;
#28093=UNCERTAINTY_MEASURE_WITH_UNIT (LENGTH_MEASURE( 1.000000000000000082E-05 ), #47359, 'distance_accuracy_value', 'NONE');
#28145=CARTESIAN_POINT ( 'NONE',  ( 3.749999999999992006, -5.946699141100872943, 19.39062500000000355 ) ) ;
#28175=CARTESIAN_POINT ( 'NONE',  ( -2.724691934501232371, -8.700186371490559623, 19.76375670625849423 ) ) ;
#28186=CARTESIAN_POINT ( 'NONE',  ( 2.775308065498768517, -8.577988221561467341, 16.79500670625849068 ) ) ;
#28193=CARTESIAN_POINT ( 'NONE',  ( -1.492201783934593573, -3.724691934501250135, 20.57999329374151998 ) ) ;
#28198=CARTESIAN_POINT ( 'NONE',  ( -1.492201783934593573, -3.724691934501250135, 21.82999329374151642 ) ) ;
#28284=CARTESIAN_POINT ( 'NONE',  ( -3.775308065498766297, -6.007798216065450170, 17.42000670625848713 ) ) ;
#28286=VERTEX_POINT ( 'NONE', #21060 ) ;
#28292=CARTESIAN_POINT ( 'NONE',  ( -1.492201783934549164, -11.27530806549876807, 15.85750670625849068 ) ) ;
#28309=CARTESIAN_POINT ( 'NONE',  ( -1.077988221561493543, -4.724691934501247914, 23.07999329374151998 ) ) ;
#28390=EDGE_CURVE ( 'NONE', #55297, #61929, #23101, .T. ) ;
#28418=CARTESIAN_POINT ( 'NONE',  ( -3.749999999999997780, -7.438900925035489387, 15.34561829374151465 ) ) ;
#28428=CARTESIAN_POINT ( 'NONE',  ( -2.749999999999998224, -7.500000000000015987, 15.09375000000000000 ) ) ;
#28532=CARTESIAN_POINT ( 'NONE',  ( 2.750000000000001776, -7.499999999999984013, 25.71875000000000000 ) ) ;
#28602=CARTESIAN_POINT ( 'NONE',  ( 2.651650429449539104, -4.848349570550432475, 23.06250000000000000 ) ) ;
#28634=CARTESIAN_POINT ( 'NONE',  ( 1.987747218494664292, -9.401340078031346081, 24.37313170625848713 ) ) ;
#28645=CARTESIAN_POINT ( 'NONE',  ( -1.987747218494660295, -5.598659921968651254, 16.24813170625848713 ) ) ;
#28652=CARTESIAN_POINT ( 'NONE',  ( -3.775308065498748977, -8.992201783934593351, 24.01749329374151287 ) ) ;
#28657=CARTESIAN_POINT ( 'NONE',  ( 2.608446859217924629, -10.19485399968118422, 23.62686829374151287 ) ) ;
#28743=CARTESIAN_POINT ( 'NONE',  ( -1.553300858899081538, -11.25000000000000711, 26.10937500000001066 ) ) ;
#28753=CARTESIAN_POINT ( 'NONE',  ( 2.651650429449569302, -10.15165042944953733, 25.87500000000000355 ) ) ;
#28769=CARTESIAN_POINT ( 'NONE',  ( 2.750000000000002665, -7.561099074964516831, 20.97061829374151642 ) ) ;
#28880=CARTESIAN_POINT ( 'NONE',  ( 1.987747218494642309, -5.598659921968629050, 24.56436829374151287 ) ) ;
#28885=EDGE_CURVE ( 'NONE', #73515, #55297, #39164, .T. ) ;
#28910=ADVANCED_FACE ( 'NONE', ( #26731 ), #23610, .T. ) ;
#28988=CARTESIAN_POINT ( 'NONE',  ( -1.409462824231155764E-14, -4.749999999999999112, 22.90625000000000355 ) ) ;
#29056=CARTESIAN_POINT ( 'NONE',  ( -2.651650429449535551, -10.15165042944956753, 23.68750000000000000 ) ) ;
#29089=CARTESIAN_POINT ( 'NONE',  ( -2.749999999999997780, -7.561099074964547917, 24.84188170625848713 ) ) ;
#29100=CARTESIAN_POINT ( 'NONE',  ( 1.077988221561464899, -4.724691934501233703, 25.23250670625849068 ) ) ;
#29107=CARTESIAN_POINT ( 'NONE',  ( 2.320192649118979489E-14, -11.25000000000000000, 16.03125000000000000 ) ) ;
#29111=CARTESIAN_POINT ( 'NONE',  ( -2.651650429449565305, -4.848349570550461785, 17.75000000000000355 ) ) ;
#29195=CARTESIAN_POINT ( 'NONE',  ( -2.608446859217889546, -10.19485399968121264, 22.18563170625848713 ) ) ;
#29203=CARTESIAN_POINT ( 'NONE',  ( 0.06109907496455496689, -11.24999999999999822, 23.27938170625849068 ) ) ;
#29218=CARTESIAN_POINT ( 'NONE',  ( -1.901340078031369618, -5.512252781505359245, 23.00186829374151287 ) ) ;
#29293=CARTESIAN_POINT ( 'NONE',  ( -1.553300858899081538, -11.25000000000000711, 18.60937500000000355 ) ) ;
#29317=CARTESIAN_POINT ( 'NONE',  ( -2.724691934501246582, -6.299813628509474128, 24.17374329374151642 ) ) ;
#29321=CARTESIAN_POINT ( 'NONE',  ( -1.944543648263014957, -5.555456351737005249, 21.50000000000000000 ) ) ;
#29427=CARTESIAN_POINT ( 'NONE',  ( -1.944543648262992530, -9.444543648263016067, 26.18750000000000355 ) ) ;
#29489=CARTESIAN_POINT ( 'NONE',  ( -1.929879867024197893E-14, -3.750000000000000000, 25.40625000000000000 ) ) ;
#29521=CARTESIAN_POINT ( 'NONE',  ( 1.077988221561464899, -4.724691934501233703, 23.98250670625849068 ) ) ;
#29532=CARTESIAN_POINT ( 'NONE',  ( 2.724691934501235036, -6.299813628509441266, 24.13875670625849068 ) ) ;
#29539=CARTESIAN_POINT ( 'NONE',  ( 3.750000000000009770, -9.053300858899081760, 14.54687500000000178 ) ) ;
#29546=CARTESIAN_POINT ( 'NONE',  ( 3.749999999999992006, -5.946699141100872943, 15.64062500000000178 ) ) ;
#29585=CARTESIAN_POINT ( 'NONE',  ( -1.929879867024197893E-14, -3.750000000000000000, 20.40625000000000000 ) ) ;
#29628=CARTESIAN_POINT ( 'NONE',  ( -1.614399933863656544, -3.775308065498769405, 22.57625670625848713 ) ) ;
#29636=CARTESIAN_POINT ( 'NONE',  ( -3.749999999999996447, -7.561099074964554134, 23.59188170625849068 ) ) ;
#29650=CARTESIAN_POINT ( 'NONE',  ( 0.06109907496451789238, -4.749999999999998224, 24.40811829374151642 ) ) ;
#29731=CARTESIAN_POINT ( 'NONE',  ( -2.651650429449535551, -10.15165042944956753, 14.93750000000000000 ) ) ;
#29741=CARTESIAN_POINT ( 'NONE',  ( -3.750000000000008438, -5.946699141100917352, 18.92187500000000355 ) ) ;
#29754=CARTESIAN_POINT ( 'NONE',  ( -1.614399933863613468, -11.22469193450124969, 15.11124329374151287 ) ) ;
#29758=CARTESIAN_POINT ( 'NONE',  ( -1.944543648263014957, -5.555456351737005249, 24.00000000000000000 ) ) ;
#29859=CARTESIAN_POINT ( 'NONE',  ( 1.139087296526029469, -10.24999999999999467, 22.20312500000000000 ) ) ;
#29931=CARTESIAN_POINT ( 'NONE',  ( 1.553300858899129722, -11.24999999999999112, 23.45312500000000000 ) ) ;
#29961=CARTESIAN_POINT ( 'NONE',  ( 1.077988221561464899, -4.724691934501233703, 20.23250670625849423 ) ) ;
#29971=CARTESIAN_POINT ( 'NONE',  ( 1.200186371490561621, -10.22469193450123193, 21.95125670625849068 ) ) ;
#29979=CARTESIAN_POINT ( 'NONE',  ( -1.553300858899081538, -11.25000000000000711, 17.35937500000000000 ) ) ;
#29986=CARTESIAN_POINT ( 'NONE',  ( -3.749999999999988454, -9.053300858899127945, 16.26562500000000000 ) ) ;
#29995=DIRECTION ( 'NONE',  ( -0.7071067811865510144, 0.7071067811865440200, 0.000000000000000000 ) ) ;
#30024=CARTESIAN_POINT ( 'NONE',  ( -3.749999999999997335, -7.500000000000021316, 22.59375000000000355 ) ) ;
#30064=CARTESIAN_POINT ( 'NONE',  ( 3.775308065498768517, -8.992201783934554271, 19.29500670625849068 ) ) ;
#30072=CARTESIAN_POINT ( 'NONE',  ( -3.749999999999996447, -7.561099074964554134, 19.84188170625848713 ) ) ;
#30088=CARTESIAN_POINT ( 'NONE',  ( -3.775308065498748977, -8.992201783934593351, 15.26749329374151465 ) ) ;
#30168=CARTESIAN_POINT ( 'NONE',  ( 3.750000000000000888, -7.499999999999978684, 14.46875000000000000 ) ) ;
#30177=CARTESIAN_POINT ( 'NONE',  ( 1.553300858899129944, -11.24999999999998934, 19.70312500000000355 ) ) ;
#30195=CARTESIAN_POINT ( 'NONE',  ( 3.750000000000001776, -7.561099074964511502, 19.72061829374151287 ) ) ;
#30200=CARTESIAN_POINT ( 'NONE',  ( -1.944543648262992530, -9.444543648263016067, 23.68750000000000000 ) ) ;
#30298=CARTESIAN_POINT ( 'NONE',  ( 1.944543648263018731, -9.444543648262994751, 24.62500000000000000 ) ) ;
#30366=CARTESIAN_POINT ( 'NONE',  ( 3.750000000000009770, -9.053300858899081760, 23.29687500000000000 ) ) ;
#30400=CARTESIAN_POINT ( 'NONE',  ( 1.901340078031349856, -5.512252781505337929, 22.81063170625848713 ) ) ;
#30403=CARTESIAN_POINT ( 'NONE',  ( 3.365693839367760010, -7.795565839780282502, 14.00000000000000178 ) ) ;
#30412=CARTESIAN_POINT ( 'NONE',  ( 1.901340078031349856, -5.512252781505337929, 21.56063170625849068 ) ) ;
#30420=CARTESIAN_POINT ( 'NONE',  ( -3.750000000000008438, -5.946699141100917352, 17.67187500000000355 ) ) ;
#30425=CARTESIAN_POINT ( 'NONE',  ( -2.651650429449565305, -4.848349570550461785, 15.25000000000000000 ) ) ;
#30458=CARTESIAN_POINT ( 'NONE',  ( -2.651650429449535551, -10.15165042944956753, 23.68750000000000000 ) ) ;
#30499=CARTESIAN_POINT ( 'NONE',  ( 2.694853999681214862, -10.10844685921789043, 21.87313170625849068 ) ) ;
#30510=CARTESIAN_POINT ( 'NONE',  ( -2.608446859217889546, -10.19485399968121264, 19.68563170625849068 ) ) ;
#30523=CARTESIAN_POINT ( 'NONE',  ( -1.614399933863613468, -11.22469193450124969, 13.86124329374151820 ) ) ;
#30598=CARTESIAN_POINT ( 'NONE',  ( -2.651650429449565305, -4.848349570550461785, 15.25000000000000000 ) ) ;
#30609=CARTESIAN_POINT ( 'NONE',  ( 3.749999999999992006, -5.946699141100872943, 15.64062500000000178 ) ) ;
#30624=CARTESIAN_POINT ( 'NONE',  ( -3.775308065498748977, -8.992201783934593351, 19.01749329374151287 ) ) ;
#30629=CARTESIAN_POINT ( 'NONE',  ( 2.749999999999995115, -6.360912703473971419, 24.39062500000000000 ) ) ;
#30635=CARTESIAN_POINT ( 'NONE',  ( -1.409462824231155764E-14, -4.749999999999999112, 20.40625000000000000 ) ) ;
#30731=CARTESIAN_POINT ( 'NONE',  ( 0.06109907496451789238, -4.749999999999998224, 13.15811829374151642 ) ) ;
#30837=CARTESIAN_POINT ( 'NONE',  ( 2.724691934501235036, -6.299813628509441266, 25.38875670625849423 ) ) ;
#30839=CARTESIAN_POINT ( 'NONE',  ( 1.337245517230120306, -4.028657149949338212, 14.00000000000000533 ) ) ;
#30846=CARTESIAN_POINT ( 'NONE',  ( -1.901340078031346525, -9.487747218494661183, 22.18563170625848713 ) ) ;
#30854=CARTESIAN_POINT ( 'NONE',  ( -1.553300858899125059, -3.750000000000009326, 17.82812500000000000 ) ) ;
#30858=CARTESIAN_POINT ( 'NONE',  ( -3.749999999999997335, -7.500000000000021316, 16.34375000000000000 ) ) ;
#30894=CARTESIAN_POINT ( 'NONE',  ( 1.553300858899129944, -11.24999999999998934, 20.95312500000000000 ) ) ;
#30931=CARTESIAN_POINT ( 'NONE',  ( -1.492201783934549164, -11.27530806549876807, 19.60750670625849068 ) ) ;
#30942=CARTESIAN_POINT ( 'NONE',  ( -2.608446859217889546, -10.19485399968121264, 22.18563170625848713 ) ) ;
#30957=CARTESIAN_POINT ( 'NONE',  ( -2.608446859217920633, -4.805146000318815780, 13.00186829374151465 ) ) ;
#31038=CARTESIAN_POINT ( 'NONE',  ( -3.749999999999988454, -9.053300858899127945, 16.26562500000000000 ) ) ;
#31048=CARTESIAN_POINT ( 'NONE',  ( -1.929879867024197893E-14, -3.750000000000000000, 16.65625000000000000 ) ) ;
#31063=CARTESIAN_POINT ( 'NONE',  ( 2.694853999681185108, -4.891553140782077591, 19.56436829374151287 ) ) ;
#31069=CARTESIAN_POINT ( 'NONE',  ( -2.750000000000007105, -6.360912703474006946, 23.92187500000000355 ) ) ;
#31075=CARTESIAN_POINT ( 'NONE',  ( 1.944543648263018731, -9.444543648262994751, 17.12500000000000000 ) ) ;
#31171=CARTESIAN_POINT ( 'NONE',  ( 0.06109907496451789238, -4.749999999999998224, 14.40811829374151110 ) ) ;
#31292=CARTESIAN_POINT ( 'NONE',  ( -2.724691934501232371, -8.700186371490559623, 26.01375670625848713 ) ) ;
#31294=CARTESIAN_POINT ( 'NONE',  ( 3.014247786467086687, -7.171217661578389801, 14.00000000000001066 ) ) ;
#31301=CARTESIAN_POINT ( 'NONE',  ( 1.139087296526029469, -10.24999999999999467, 15.95312500000000000 ) ) ;
#31311=CARTESIAN_POINT ( 'NONE',  ( 3.750000000000000888, -7.499999999999978684, 20.71875000000000000 ) ) ;
#31353=CARTESIAN_POINT ( 'NONE',  ( 2.651650429449539104, -4.848349570550432475, 23.06250000000000000 ) ) ;
#31360=CARTESIAN_POINT ( 'NONE',  ( 3.750000000000000888, -7.499999999999978684, 15.71875000000000000 ) ) ;
#31392=CARTESIAN_POINT ( 'NONE',  ( 3.775308065498768517, -8.992201783934554271, 26.79500670625849423 ) ) ;
#31401=CARTESIAN_POINT ( 'NONE',  ( 3.775308065498768517, -8.992201783934554271, 24.29500670625849423 ) ) ;
#31416=CARTESIAN_POINT ( 'NONE',  ( 2.608446859217924629, -10.19485399968118422, 13.62686829374151642 ) ) ;
#31498=CARTESIAN_POINT ( 'NONE',  ( 2.651650429449569302, -10.15165042944953733, 20.87500000000000000 ) ) ;
#31506=CARTESIAN_POINT ( 'NONE',  ( -3.750000000000008438, -5.946699141100917352, 17.67187500000000355 ) ) ;
#31526=CARTESIAN_POINT ( 'NONE',  ( 1.944543648263018731, -9.444543648262994751, 24.62500000000000000 ) ) ;
#31533=CARTESIAN_POINT ( 'NONE',  ( 1.944543648262996083, -5.555456351736983045, 20.56250000000000000 ) ) ;
#31629=CARTESIAN_POINT ( 'NONE',  ( -1.077988221561493543, -4.724691934501247914, 16.82999329374151287 ) ) ;
#31743=CARTESIAN_POINT ( 'NONE',  ( 1.944543648263018731, -9.444543648262994751, 15.87500000000000000 ) ) ;
#31754=CARTESIAN_POINT ( 'NONE',  ( -1.944543648263014957, -5.555456351737005249, 16.50000000000000000 ) ) ;
#31765=CARTESIAN_POINT ( 'NONE',  ( 1.553300858899087311, -3.749999999999992006, 20.48437500000000000 ) ) ;
#31806=CARTESIAN_POINT ( 'NONE',  ( -3.750000000000008438, -5.946699141100917352, 25.17187500000000000 ) ) ;
#31816=CARTESIAN_POINT ( 'NONE',  ( 3.749999999999992006, -5.946699141100872943, 16.89062500000000000 ) ) ;
#31846=CARTESIAN_POINT ( 'NONE',  ( -2.608446859217889546, -10.19485399968121264, 24.68563170625849068 ) ) ;
#31856=CARTESIAN_POINT ( 'NONE',  ( -2.694853999681210865, -4.891553140782108677, 26.24813170625849068 ) ) ;
#31870=CARTESIAN_POINT ( 'NONE',  ( -2.608446859217920633, -4.805146000318815780, 16.75186829374151287 ) ) ;
#31951=CARTESIAN_POINT ( 'NONE',  ( -3.749999999999997335, -7.500000000000021316, 22.59375000000000355 ) ) ;
#31959=CARTESIAN_POINT ( 'NONE',  ( 2.651650429449569302, -10.15165042944953733, 24.62500000000000000 ) ) ;
#31977=CARTESIAN_POINT ( 'NONE',  ( 0.06109907496451789238, -4.749999999999998224, 14.40811829374151110 ) ) ;
#31982=CARTESIAN_POINT ( 'NONE',  ( -2.749999999999998224, -7.500000000000015987, 20.09375000000000000 ) ) ;
#32073=CARTESIAN_POINT ( 'NONE',  ( -2.749999999999999112, -7.438900925035484057, 17.84561829374150932 ) ) ;
#32186=CARTESIAN_POINT ( 'NONE',  ( 0.06109907496454976272, -10.25000000000000000, 25.77938170625848713 ) ) ;
#32199=CARTESIAN_POINT ( 'NONE',  ( 2.775308065498768517, -8.577988221561467341, 26.79500670625849423 ) ) ;
#32209=CARTESIAN_POINT ( 'NONE',  ( -3.749999999999997335, -7.500000000000021316, 23.84375000000000000 ) ) ;
#32257=CARTESIAN_POINT ( 'NONE',  ( -3.750000000000007550, -5.946699141100917352, 17.67187500000000355 ) ) ;
#32286=CARTESIAN_POINT ( 'NONE',  ( 1.614399933863660985, -11.22469193450123193, 26.95125670625849068 ) ) ;
#32296=CARTESIAN_POINT ( 'NONE',  ( 1.200186371490561621, -10.22469193450123193, 15.70125670625848890 ) ) ;
#32311=CARTESIAN_POINT ( 'NONE',  ( -0.06109907496450878162, -11.25000000000000000, 18.78311829374151287 ) ) ;
#32390=CARTESIAN_POINT ( 'NONE',  ( -3.749999999999997335, -7.500000000000021316, 21.34375000000000000 ) ) ;
#32400=CARTESIAN_POINT ( 'NONE',  ( -1.553300858899081538, -11.25000000000000711, 24.85937500000001421 ) ) ;
#32416=CARTESIAN_POINT ( 'NONE',  ( -2.775308065498752086, -8.577988221561495763, 16.51749329374151642 ) ) ;
#32421=CARTESIAN_POINT ( 'NONE',  ( -1.139087296526025250, -4.750000000000006217, 16.57812500000000000 ) ) ;
#32509=CARTESIAN_POINT ( 'NONE',  ( -1.077988221561493543, -4.724691934501247914, 15.57999329374151110 ) ) ;
#32535=( NAMED_UNIT ( * ) SI_UNIT ( $, .STERADIAN. ) SOLID_ANGLE_UNIT ( ) );
#32620=CARTESIAN_POINT ( 'NONE',  ( 2.775308065498768517, -8.577988221561467341, 25.54500670625849779 ) ) ;
#32630=CARTESIAN_POINT ( 'NONE',  ( -1.944543648263014957, -5.555456351737005249, 14.00000000000000000 ) ) ;
#32638=CARTESIAN_POINT ( 'NONE',  ( 1.553300858899129944, -11.24999999999998934, 22.20312500000000000 ) ) ;
#32680=CARTESIAN_POINT ( 'NONE',  ( 3.750000000000009770, -9.053300858899081760, 25.79687500000000355 ) ) ;
#32719=CARTESIAN_POINT ( 'NONE',  ( 2.694853999681214862, -10.10844685921789043, 23.12313170625848713 ) ) ;
#32731=CARTESIAN_POINT ( 'NONE',  ( 1.614399933863660985, -11.22469193450123193, 25.70125670625848713 ) ) ;
#32738=CARTESIAN_POINT ( 'NONE',  ( 2.694853999681185108, -4.891553140782077591, 15.81436829374151465 ) ) ;
#32746=CARTESIAN_POINT ( 'NONE',  ( -3.749999999999997780, -7.438900925035489387, 17.84561829374150932 ) ) ;
#32834=CARTESIAN_POINT ( 'NONE',  ( -2.651650429449535551, -10.15165042944956753, 19.93750000000000000 ) ) ;
#32837=( BOUNDED_CURVE ( )  B_SPLINE_CURVE ( 2, ( #71178, #77498, #36946, #83833, #70749, #1842, #21222, #63086, #36524, #56779, #956, #7725, #35185, #49140, #28428, #21672, #69860, #22116, #15812, #63971, #35638, #64409, #63535, #84279, #42837, #70302, #22556, #2267, #57229, #84722, #58107, #50888, #25220, #32421, #80172, #51777, #4956, #85589, #66198, #52682, #31075, #79280, #10377, #18471, #45925, #59447, #86039, #71617, #37387, #44580, #37840, #23865, #73414, #72066, #78376, #58996, #4504, #72962, #16680, #11718, #39193, #38292, #4043, #65747, #3158, #17582, #44136, #66654, #3606, #11263, #51320, #64856, #38736, #85150, #9923, #78823, #23433, #45032, #31982, #58542, #24316, #86952, #30635, #17123, #31533, #65308, #72510, #10821, #86497, #24771, #52236, #79726, #18026, #45483, #20244, #33318, #46382, #54014, #60330, #87843, #60776, #47706, #40525, #68862, #12600, #81953, #6291, #12159, #80628, #7169, #26109, #18910, #73863, #5842, #19353, #39641, #26560, #81508, #13480, #88285, #59889, #67991, #67543, #75192, #61211, #46821, #40088, #33754, #87385, #68421, #74299, #19796, #47259, #74751, #61655, #53123, #67101, #25667, #40956, #5402, #89161, #32868, #53574, #13040, #88721, #81069, #26999, #54457, #6719, #34191, #27441, #54909, #82392, #20678, #48142, #75612, #13918, #41400, #35975, #43601, #7614 ),
 .UNSPECIFIED., .F., .F. ) 
 B_SPLINE_CURVE_WITH_KNOTS ( ( 3, 2, 2, 2, 2, 2, 2, 2, 2, 2, 2, 2, 2, 2, 2, 2, 2, 2, 2, 2, 2, 2, 2, 2, 2, 2, 2, 2, 2, 2, 2, 2, 2, 2, 2, 2, 2, 2, 2, 2, 2, 2, 2, 2, 2, 2, 2, 2, 2, 2, 2, 2, 2, 2, 2, 2, 2, 2, 2, 2, 2, 2, 2, 2, 2, 2, 2, 2, 2, 2, 2, 2, 2, 2, 2, 2, 2, 2, 2, 2, 3 ),
 ( 0.000000000000000000, 0.01250000000000000069, 0.02500000000000000139, 0.03749999999999999861, 0.05000000000000000278, 0.06250000000000000000, 0.07499999999999999722, 0.08749999999999999445, 0.1000000000000000056, 0.1125000000000000028, 0.1250000000000000000, 0.1375000000000000111, 0.1499999999999999944, 0.1625000000000000056, 0.1749999999999999889, 0.1875000000000000000, 0.2000000000000000111, 0.2124999999999999944, 0.2250000000000000056, 0.2374999999999999889, 0.2500000000000000000, 0.2625000000000000111, 0.2750000000000000222, 0.2874999999999999778, 0.2999999999999999889, 0.3125000000000000000, 0.3250000000000000111, 0.3375000000000000222, 0.3499999999999999778, 0.3624999999999999889, 0.3750000000000000000, 0.3875000000000000111, 0.4000000000000000222, 0.4124999999999999778, 0.4249999999999999889, 0.4375000000000000000, 0.4500000000000000111, 0.4625000000000000222, 0.4749999999999999778, 0.4874999999999999889, 0.5000000000000000000, 0.5124999999999999556, 0.5250000000000000222, 0.5374999999999999778, 0.5500000000000000444, 0.5625000000000000000, 0.5749999999999999556, 0.5875000000000000222, 0.5999999999999999778, 0.6125000000000000444, 0.6250000000000000000, 0.6374999999999999556, 0.6500000000000000222, 0.6624999999999999778, 0.6750000000000000444, 0.6875000000000000000, 0.6999999999999999556, 0.7125000000000000222, 0.7249999999999999778, 0.7375000000000000444, 0.7500000000000000000, 0.7624999999999999556, 0.7750000000000000222, 0.7874999999999999778, 0.8000000000000000444, 0.8125000000000000000, 0.8249999999999999556, 0.8375000000000000222, 0.8499999999999999778, 0.8625000000000000444, 0.8750000000000000000, 0.8874999999999999556, 0.9000000000000000222, 0.9124999999999999778, 0.9250000000000000444, 0.9375000000000000000, 0.9499999999999999556, 0.9625000000000000222, 0.9749999999999999778, 0.9875000000000000444, 1.000000000000000000 ),
 .UNSPECIFIED. ) 
 CURVE ( )  GEOMETRIC_REPRESENTATION_ITEM ( )  RATIONAL_B_SPLINE_CURVE ( ( 1.000000000000000000, 0.9238795325112867385, 1.000000000000000000, 0.9238795325112867385, 1.000000000000000000, 0.9238795325112867385, 1.000000000000000000, 0.9238795325112867385, 1.000000000000000000, 0.9238795325112867385, 1.000000000000000000, 0.9238795325112867385, 1.000000000000000000, 0.9238795325112867385, 1.000000000000000000, 0.9238795325112867385, 1.000000000000000000, 0.9238795325112867385, 1.000000000000000000, 0.9238795325112867385, 1.000000000000000000, 0.9238795325112867385, 1.000000000000000000, 0.9238795325112867385, 1.000000000000000000, 0.9238795325112867385, 1.000000000000000000, 0.9238795325112867385, 1.000000000000000000, 0.9238795325112867385, 1.000000000000000000, 0.9238795325112867385, 1.000000000000000000, 0.9238795325112867385, 1.000000000000000000, 0.9238795325112867385, 1.000000000000000000, 0.9238795325112867385, 1.000000000000000000, 0.9238795325112867385, 1.000000000000000000, 0.9238795325112867385, 1.000000000000000000, 0.9238795325112867385, 1.000000000000000000, 0.9238795325112867385, 1.000000000000000000, 0.9238795325112867385, 1.000000000000000000, 0.9238795325112867385, 1.000000000000000000, 0.9238795325112867385, 1.000000000000000000, 0.9238795325112867385, 1.000000000000000000, 0.9238795325112867385, 1.000000000000000000, 0.9238795325112867385, 1.000000000000000000, 0.9238795325112867385, 1.000000000000000000, 0.9238795325112867385, 1.000000000000000000, 0.9238795325112867385, 1.000000000000000000, 0.9238795325112867385, 1.000000000000000000, 0.9238795325112867385, 1.000000000000000000, 0.9238795325112867385, 1.000000000000000000, 0.9238795325112867385, 1.000000000000000000, 0.9238795325112867385, 1.000000000000000000, 0.9238795325112867385, 1.000000000000000000, 0.9238795325112867385, 1.000000000000000000, 0.9238795325112867385, 1.000000000000000000, 0.9238795325112867385, 1.000000000000000000, 0.9238795325112867385, 1.000000000000000000, 0.9238795325112867385, 1.000000000000000000, 0.9238795325112867385, 1.000000000000000000, 0.9238795325112867385, 1.000000000000000000, 0.9238795325112867385, 1.000000000000000000, 0.9238795325112867385, 1.000000000000000000, 0.9238795325112867385, 1.000000000000000000, 0.9238795325112867385, 1.000000000000000000, 0.9238795325112867385, 1.000000000000000000, 0.9238795325112867385, 1.000000000000000000, 0.9238795325112867385, 1.000000000000000000, 0.9238795325112867385, 1.000000000000000000, 0.9238795325112867385, 1.000000000000000000, 0.9238795325112867385, 1.000000000000000000, 0.9238795325112867385, 1.000000000000000000, 0.9238795325112867385, 1.000000000000000000, 0.9238795325112867385, 1.000000000000000000, 0.9238795325112867385, 1.000000000000000000, 0.9238795325112867385, 1.000000000000000000, 0.9238795325112867385, 1.000000000000000000, 0.9238795325112867385, 1.000000000000000000, 0.9238795325112867385, 1.000000000000000000, 0.9238795325112867385, 1.000000000000000000, 0.9238795325112867385, 1.000000000000000000, 0.9238795325112867385, 1.000000000000000000, 0.9238795325112867385, 1.000000000000000000, 0.9238795325112867385, 1.000000000000000000, 0.9238795325112867385, 1.000000000000000000, 0.9238795325112867385, 1.000000000000000000, 0.9238795325112867385, 1.000000000000000000, 0.9238795325112867385, 1.000000000000000000, 0.9238795325112867385, 1.000000000000000000, 0.9238795325112867385, 1.000000000000000000, 0.9238795325112867385, 1.000000000000000000, 0.9238795325112867385, 1.000000000000000000, 0.9238795325112867385, 1.000000000000000000, 0.9238795325112867385, 1.000000000000000000, 0.9238795325112867385, 1.000000000000000000, 0.9238795325112867385, 1.000000000000000000 ) ) 
 REPRESENTATION_ITEM ( '' )  );
#32844=CARTESIAN_POINT ( 'NONE',  ( 3.750000000000009770, -9.053300858899081760, 23.29687500000000000 ) ) ;
#32860=CARTESIAN_POINT ( 'NONE',  ( 1.901340078031373171, -9.487747218494639867, 14.87686829374151465 ) ) ;
#32868=CARTESIAN_POINT ( 'NONE',  ( -2.749999999999991562, -8.639087296526026805, 25.01562500000000000 ) ) ;
#32964=CARTESIAN_POINT ( 'NONE',  ( -0.06109907496451398579, -10.25000000000000178, 21.28311829374151287 ) ) ;
#33069=CARTESIAN_POINT ( 'NONE',  ( -1.139087296525992166, -10.25000000000000533, 17.35937500000000000 ) ) ;
#33077=CARTESIAN_POINT ( 'NONE',  ( -2.724691934501232371, -8.700186371490559623, 27.26375670625849423 ) ) ;
#33085=CARTESIAN_POINT ( 'NONE',  ( -1.929879867024197893E-14, -3.750000000000000000, 19.15625000000000000 ) ) ;
#33133=CARTESIAN_POINT ( 'NONE',  ( 3.750000000000009770, -9.053300858899081760, 18.29687500000000000 ) ) ;
#33167=CARTESIAN_POINT ( 'NONE',  ( 1.614399933863660985, -11.22469193450123193, 25.70125670625848713 ) ) ;
#33180=CARTESIAN_POINT ( 'NONE',  ( 1.492201783934554493, -3.724691934501233703, 26.48250670625848713 ) ) ;
#33187=CARTESIAN_POINT ( 'NONE',  ( -1.492201783934593573, -3.724691934501250135, 15.57999329374151110 ) ) ;
#33194=CARTESIAN_POINT ( 'NONE',  ( 2.694853999681185108, -4.891553140782077591, 18.31436829374150932 ) ) ;
#33285=CARTESIAN_POINT ( 'NONE',  ( -1.553300858899081538, -11.25000000000000711, 22.35937500000000711 ) ) ;
#33295=CARTESIAN_POINT ( 'NONE',  ( 2.651650429449539104, -4.848349570550432475, 21.81250000000000000 ) ) ;
#33311=CARTESIAN_POINT ( 'NONE',  ( 1.901340078031373171, -9.487747218494639867, 17.37686829374151287 ) ) ;
#33318=CARTESIAN_POINT ( 'NONE',  ( -2.750000000000006217, -6.360912703474006946, 21.42187500000000000 ) ) ;
#33412=CARTESIAN_POINT ( 'NONE',  ( -1.077988221561493543, -4.724691934501247914, 20.57999329374151998 ) ) ;
#33521=CARTESIAN_POINT ( 'NONE',  ( 1.944543648262996083, -5.555456351736983045, 18.06250000000000355 ) ) ;
#33531=CARTESIAN_POINT ( 'NONE',  ( 1.799775606325937360E-14, -10.25000000000000000, 19.78125000000000000 ) ) ;
#33587=CARTESIAN_POINT ( 'NONE',  ( -1.553300858899125059, -3.750000000000009326, 22.82812500000000355 ) ) ;
#33614=CARTESIAN_POINT ( 'NONE',  ( 2.750000000000001332, -7.438900925035452083, 17.96688170625848713 ) ) ;
#33627=CARTESIAN_POINT ( 'NONE',  ( -2.724691934501232371, -8.700186371490559623, 17.26375670625849068 ) ) ;
#33634=CARTESIAN_POINT ( 'NONE',  ( 3.724691934501251023, -9.114399933863618131, 23.54874329374151642 ) ) ;
#33640=CARTESIAN_POINT ( 'NONE',  ( -1.492201783934593573, -3.724691934501250135, 19.32999329374151642 ) ) ;
#33722=CARTESIAN_POINT ( 'NONE',  ( 3.724691934501232815, -5.885600066136343678, 16.63875670625849068 ) ) ;
#33733=CARTESIAN_POINT ( 'NONE',  ( 2.320192649118979489E-14, -11.25000000000000000, 22.28125000000000355 ) ) ;
#33747=CARTESIAN_POINT ( 'NONE',  ( 1.077988221561497539, -10.27530806549875386, 17.45499329374151642 ) ) ;
#33754=CARTESIAN_POINT ( 'NONE',  ( -2.750000000000006217, -6.360912703474006946, 23.92187500000000355 ) ) ;
#33845=CARTESIAN_POINT ( 'NONE',  ( -1.200186371490524317, -10.22469193450124791, 22.61124329374151287 ) ) ;
#33951=CARTESIAN_POINT ( 'NONE',  ( 2.750000000000008438, -8.639087296525996607, 19.54687499999999645 ) ) ;
#33959=CARTESIAN_POINT ( 'NONE',  ( 1.139087296526029469, -10.24999999999999467, 22.20312500000000000 ) ) ;
#33966=CARTESIAN_POINT ( 'NONE',  ( 3.750000000000009770, -9.053300858899081760, 25.79687500000000355 ) ) ;
#34018=CARTESIAN_POINT ( 'NONE',  ( -2.651650429449535551, -10.15165042944956753, 22.43750000000000000 ) ) ;
#34051=CARTESIAN_POINT ( 'NONE',  ( 1.901340078031349856, -5.512252781505337929, 15.31063170625849068 ) ) ;
#34064=CARTESIAN_POINT ( 'NONE',  ( 2.750000000000001332, -7.438900925035452083, 19.21688170625848358 ) ) ;
#34072=CARTESIAN_POINT ( 'NONE',  ( -3.724691934501248802, -5.885600066136383646, 24.17374329374151642 ) ) ;
#34077=CARTESIAN_POINT ( 'NONE',  ( -3.724691934501248802, -5.885600066136383646, 25.42374329374151998 ) ) ;
#34159=CARTESIAN_POINT ( 'NONE',  ( -3.749999999999997335, -7.500000000000021316, 25.09374999999999645 ) ) ;
#34168=CARTESIAN_POINT ( 'NONE',  ( 1.614399933863660985, -11.22469193450123193, 18.20125670625849068 ) ) ;
#34183=CARTESIAN_POINT ( 'NONE',  ( -0.06109907496451398579, -10.25000000000000178, 23.78311829374151998 ) ) ;
#34191=CARTESIAN_POINT ( 'NONE',  ( 2.749999999999995115, -6.360912703473971419, 25.64062500000000000 ) ) ;
#34287=CARTESIAN_POINT ( 'NONE',  ( -2.724691934501246582, -6.299813628509474128, 22.92374329374151998 ) ) ;
#34340=CARTESIAN_POINT ( 'NONE',  ( 3.749999999999992006, -5.946699141100872943, 25.64062500000000000 ) ) ;
#34393=CARTESIAN_POINT ( 'NONE',  ( -1.139087296526025916, -4.750000000000006217, 19.07812500000000000 ) ) ;
#34402=CARTESIAN_POINT ( 'NONE',  ( -2.749999999999998224, -7.500000000000015987, 18.84375000000000000 ) ) ;
#34409=CARTESIAN_POINT ( 'NONE',  ( -1.929879867024197893E-14, -3.750000000000000000, 24.15625000000000000 ) ) ;
#34464=CARTESIAN_POINT ( 'NONE',  ( 1.553300858899086867, -3.749999999999992006, 21.73437500000000000 ) ) ;
#34496=CARTESIAN_POINT ( 'NONE',  ( -2.724691934501232371, -8.700186371490559623, 18.51375670625849068 ) ) ;
#34509=CARTESIAN_POINT ( 'NONE',  ( -1.987747218494660295, -5.598659921968651254, 17.49813170625848713 ) ) ;
#34517=( GEOMETRIC_REPRESENTATION_CONTEXT ( 3 ) GLOBAL_UNCERTAINTY_ASSIGNED_CONTEXT ( ( #57234 ) ) GLOBAL_UNIT_ASSIGNED_CONTEXT ( ( #25788, #25340, #87511 ) ) REPRESENTATION_CONTEXT ( 'NONE', 'WORKASPACE' ) );
#34518=CARTESIAN_POINT ( 'NONE',  ( 2.608446859217924629, -10.19485399968118422, 21.12686829374151287 ) ) ;
#34523=CARTESIAN_POINT ( 'NONE',  ( 3.749999999999992006, -5.946699141100872943, 14.39062500000000178 ) ) ;
#34562=VECTOR ( 'NONE', #81706, 999.9999999999998863 ) ;
#34608=CARTESIAN_POINT ( 'NONE',  ( -3.775308065498766297, -6.007798216065450170, 16.17000670625848713 ) ) ;
#34616=CARTESIAN_POINT ( 'NONE',  ( 2.694853999681214862, -10.10844685921789043, 18.12313170625849068 ) ) ;
#34631=CARTESIAN_POINT ( 'NONE',  ( 2.775308065498755195, -6.422011778438505125, 19.64249329374151642 ) ) ;
#34734=CARTESIAN_POINT ( 'NONE',  ( -2.749999999999999112, -7.438900925035484057, 19.09561829374150932 ) ) ;
#34784=CARTESIAN_POINT ( 'NONE',  ( 2.651650429449539104, -4.848349570550432475, 25.56250000000000355 ) ) ;
#34834=CARTESIAN_POINT ( 'NONE',  ( -2.750000000000007105, -6.360912703474006946, 17.67187500000000355 ) ) ;
#34881=CIRCLE ( 'NONE', #7568, 0.4999999999999994449 ) ;
#34900=CARTESIAN_POINT ( 'NONE',  ( 2.651650429449569302, -10.15165042944953733, 22.12500000000000000 ) ) ;
#34927=PLANE ( 'NONE',  #83260 ) ;
#34930=CARTESIAN_POINT ( 'NONE',  ( -0.06109907496454585613, -4.750000000000000000, 17.65438170625849068 ) ) ;
#34943=CARTESIAN_POINT ( 'NONE',  ( -1.077988221561460236, -10.27530806549876452, 18.35750670625849068 ) ) ;
#34953=CARTESIAN_POINT ( 'NONE',  ( -1.492201783934593573, -3.724691934501250135, 21.82999329374151642 ) ) ;
#34959=CARTESIAN_POINT ( 'NONE',  ( -2.694853999681181556, -10.10844685921792241, 21.43936829374151642 ) ) ;
#35044=CARTESIAN_POINT ( 'NONE',  ( -2.608446859217889546, -10.19485399968121264, 15.93563170625849068 ) ) ;
#35052=CARTESIAN_POINT ( 'NONE',  ( 3.724691934501232815, -5.885600066136343678, 15.38875670625848890 ) ) ;
#35068=CARTESIAN_POINT ( 'NONE',  ( 1.901340078031373171, -9.487747218494639867, 22.37686829374150932 ) ) ;
#35177=CARTESIAN_POINT ( 'NONE',  ( 2.724691934501250135, -8.700186371490531201, 23.54874329374151642 ) ) ;
#35185=CARTESIAN_POINT ( 'NONE',  ( -1.944543648262992530, -9.444543648263016067, 14.93750000000000000 ) ) ;
#35282=CARTESIAN_POINT ( 'NONE',  ( 1.139087296525997273, -4.749999999999992895, 25.48437500000000000 ) ) ;
#35298=CARTESIAN_POINT ( 'NONE',  ( -1.553300858899081538, -11.25000000000000711, 26.10937500000001066 ) ) ;
#35307=DIRECTION ( 'NONE',  ( 1.000000000000000000, 0.000000000000000000, 0.000000000000000000 ) ) ;
#35380=CARTESIAN_POINT ( 'NONE',  ( -0.06109907496454585613, -4.750000000000000000, 16.40438170625849068 ) ) ;
#35383=CARTESIAN_POINT ( 'NONE',  ( -1.399447498061196837, -4.021041001012671146, 14.00000000000000711 ) ) ;
#35393=CARTESIAN_POINT ( 'NONE',  ( 0.06109907496454976272, -10.25000000000000000, 19.52938170625848713 ) ) ;
#35400=CARTESIAN_POINT ( 'NONE',  ( 1.492201783934598236, -11.27530806549875031, 23.70499329374151642 ) ) ;
#35405=CARTESIAN_POINT ( 'NONE',  ( -3.775308065498748977, -8.992201783934593351, 21.51749329374151998 ) ) ;
#35492=CARTESIAN_POINT ( 'NONE',  ( -2.651650429449565305, -4.848349570550461785, 26.50000000000000355 ) ) ;
#35503=CARTESIAN_POINT ( 'NONE',  ( 3.749999999999999556, -7.438900925035446754, 15.46688170625848713 ) ) ;
#35520=CARTESIAN_POINT ( 'NONE',  ( 2.724691934501250135, -8.700186371490531201, 19.79874329374151287 ) ) ;
#35631=CARTESIAN_POINT ( 'NONE',  ( -2.749999999999999112, -7.438900925035484057, 25.34561829374151642 ) ) ;
#35638=CARTESIAN_POINT ( 'NONE',  ( 1.944543648262996083, -5.555456351736983045, 15.56250000000000000 ) ) ;
#35738=CARTESIAN_POINT ( 'NONE',  ( 2.749999999999995115, -6.360912703473971419, 24.39062500000000000 ) ) ;
#35742=( BOUNDED_SURFACE ( )  B_SPLINE_SURFACE ( 3, 2, ( 
 ( #933, #41929, #20758, #493, #69397, #63513, #7252, #82916, #1815, #49, #48224, #14002, #68943, #62186, #55430, #21199, #7701, #15787, #72486, #16219, #9461, #30609, #22533, #79254, #43252, #10794, #17100, #63950, #85565, #78798, #9030, #50865, #2245, #65283, #31048, #58082, #2686, #23839, #58516, #3579, #50435, #51293, #44554, #72040, #10349, #17554, #4019, #31506, #77914, #43685, #16651, #37815, #45004, #3133, #86010, #57644, #38265, #24291, #51751, #65723, #58972, #49997, #77477, #29741, #70726, #71154, #36499, #23407, #84695, #57205, #36924, #22970, #64387, #30177, #85127, #78351, #44113, #71591, #9900, #37362, #64829, #53550, #74277, #24747, #18001, #40503, #74727, #87363, #19333, #38710, #52658, #6267, #40062, #87817, #81488, #25642, #67965, #18446, #45456, #52211, #33295, #46354, #86930, #81043, #11693, #73841, #33733, #66631, #25194, #39171, #53098, #26086, #46800, #19774, #12577, #80145, #67521, #5818, #18887, #32844, #86475, #4482, #4935, #45901, #79700, #60753, #12139, #47235, #13016, #72937, #39618, #80601, #88261, #67077, #11239, #66170, #31959, #59423, #73387, #32400, #59865, #5375, #60308, #26537, #53996, #62950, #8033, #54435, #75170, #27856, #61634, #20654, #28753, #42271, #89139, #61187, #76038, #69290, #41825, #88699, #13896 ),
 ( #13452, #14795, #69728, #7591, #41377, #35052, #35503, #1262, #27416, #62512, #828, #28292, #49013, #56215, #42709, #70172, #54888, #82370, #55323, #55763, #83705, #83252, #21539, #7145, #76934, #21988, #49461, #76491, #15237, #8479, #68398, #26980, #81930, #40935, #48119, #14341, #20220, #68840, #6696, #47684, #34616, #34168, #75590, #62082, #392, #82814, #21086, #48558, #71938, #57978, #44902, #63406, #15679, #84589, #10249, #43579, #8924, #22860, #37708, #37258, #30510, #78702, #30072, #22426, #51194, #16998, #85459, #71488, #72377, #9796, #58410, #36824, #43146, #1714, #64726, #84150, #49891, #24191, #9366, #70615, #85905, #23742, #57535, #85023, #44448, #65175, #16550, #77807, #23304, #77370, #3474, #50762, #30942, #71052, #3026, #78248, #64281, #36390, #16114, #2582, #51643, #50326, #44017, #79146, #17447, #35951, #29203, #63852, #2151, #56656, #29636, #57093, #3915, #60642, #4374, #86820, #18784, #10690, #67411, #31401, #88155, #5265, #52107, #73740, #66971, #86370, #39065, #79596, #53440, #19227, #46251, #80036, #12033, #46691, #80942, #38606, #39509, #32731, #60200, #87701, #5707, #81380, #19663, #66062, #31856, #4826, #25975, #33180, #80488, #74169, #45798, #26428, #12466, #11583, #39951, #25537, #58869, #53893, #24642, #52990, #47124 ),
 ( #38156, #59314, #65613, #17893, #25087, #45350, #72820, #11128, #52551, #32296, #18335, #73280, #66525, #59761, #87256, #6154, #28645, #62844, #75489, #7489, #26869, #40829, #83603, #28186, #75938, #69619, #13790, #56109, #6598, #33627, #40395, #21436, #34509, #75064, #69182, #89033, #61972, #21881, #54772, #13349, #27309, #41273, #14237, #34943, #7927, #62406, #68294, #55655, #41712, #7033, #20981, #74614, #81821, #82263, #34064, #12904, #722, #281, #35393, #1163, #67853, #27748, #68737, #48905, #55219, #61089, #88598, #54327, #20110, #47573, #61526, #20550, #48012, #82709, #83146, #48452, #76377, #14684, #42166, #63304, #16014, #49789, #8818, #16895, #30412, #77265, #49357, #64178, #57430, #29971, #76834, #2049, #30846, #15574, #58316, #23646, #50220, #84926, #51097, #70513, #2481, #23207, #36290, #50668, #65069, #35846, #78151, #36724, #85809, #2922, #43040, #15131, #63747, #77706, #84044, #56555, #56989, #29532, #3375, #16452, #43921, #44347, #71834, #42605, #71385, #43482, #85362, #9691, #70065, #8373, #1612, #29100, #22324, #84481, #22757, #70955, #9265, #37160, #64620, #78592, #10141, #57877, #37605, #79936, #24534, #72722, #80841, #5162, #52001, #24090, #38962, #32199, #4725, #51539, #65963, #5608, #79495, #33077, #87601, #24983, #59656 ),
 ( #32630, #60100, #17797, #87156, #25434, #52891, #11931, #19124, #60545, #79040, #45249, #11034, #18238, #80391, #46595, #18688, #46153, #59211, #39846, #66867, #25879, #53341, #73639, #74074, #39409, #31301, #12368, #67312, #38057, #38507, #66420, #17341, #31754, #58767, #44798, #86717, #72278, #86265, #10591, #65521, #3822, #4269, #52449, #45699, #73181, #11478, #26321, #67754, #47466, #63530, #6498, #60989, #74964, #1834, #179, #82615, #41611, #82161, #74509, #14134, #70298, #20884, #34402, #36518, #61864, #22551, #88935, #6057, #53788, #27646, #47023, #12805, #77494, #61425, #33531, #50019, #48355, #55118, #84273, #27206, #70745, #20002, #19560, #81277, #36079, #47914, #88491, #75832, #13252, #75396, #9047, #68199, #26764, #40733, #54663, #8605, #29321, #15806, #56775, #54223, #43271, #88060, #20453, #40291, #81718, #33959, #13690, #41168, #68634, #6931, #78818, #58989, #86492, #72956, #51313, #3153, #10814, #17119, #45477, #63967, #11257, #84718, #57225, #18020, #30200, #2263, #37381, #31069, #29758, #65740, #38286, #22989, #77934, #30629, #64404, #23426, #31526, #45026, #2703, #50454, #44573, #72061, #10373, #16237, #16672, #43702, #57664, #71172, #4037, #64852, #37833, #24766, #85146, #65303, #3600, #50884, #58535, #79721, #9477, #86032, #24311 ),
 ( #58102, #36941, #85585, #51771, #79275, #78371, #44131, #71612, #17576, #72504, #9919, #23860, #52229, #39635, #11711, #20236, #66647, #40518, #31977, #25661, #26993, #60769, #73405, #59440, #32860, #59885, #53116, #5833, #26552, #66189, #86947, #81947, #54451, #67094, #88276, #80165, #4951, #47699, #81502, #47253, #46815, #18904, #74293, #74745, #19788, #32416, #12593, #40082, #67536, #54009, #6282, #75185, #38729, #87378, #80620, #60323, #33311, #33747, #19348, #13031, #73857, #4499, #67983, #61202, #88714, #25215, #52676, #18465, #45919, #39188, #46374, #12154, #5395, #53567, #87834, #26103, #81060, #76505, #48573, #42725, #48135, #56231, #13471, #40949, #75605, #34631, #49476, #35520, #22441, #68414, #82385, #62099, #76948, #21102, #13911, #407, #15252, #14811, #8050, #83719, #7607, #89155, #28769, #22003, #62967, #49027, #49906, #42287, #35966, #14354, #20669, #6711, #69743, #61649, #27434, #1729, #76054, #41391, #63422, #1279, #35068, #62527, #70185, #8494, #83269, #55338, #843, #54903, #29218, #28309, #56670, #41840, #84163, #55777, #69308, #68856, #82829, #21555, #34183, #27871, #7162, #65189, #65626, #58883, #43160, #22876, #29650, #85921, #3042, #57111, #70630, #38169, #71068, #64297, #85473, #77384, #44917, #8937, #3929, #71952, #84604 ),
 ( #30957, #58425, #24203, #78716, #51661, #57994, #50340, #79160, #31416, #2163, #16128, #30523, #86385, #85039, #77821, #51208, #23319, #17461, #43594, #72391, #15694, #36408, #9378, #36837, #10703, #10263, #24655, #63866, #2598, #30088, #57550, #50776, #78262, #16564, #44030, #17012, #37723, #71503, #9809, #37275, #3487, #64740, #23755, #44463, #88610, #87720, #74629, #53004, #31870, #17906, #25991, #11143, #66078, #40410, #25550, #86836, #12921, #74182, #46266, #12050, #12483, #67425, #32746, #4839, #39524, #38619, #5721, #66987, #33194, #87270, #19242, #5280, #80504, #59327, #32311, #18798, #67867, #11598, #73756, #39966, #6168, #33640, #45362, #25101, #4387, #60657, #60214, #52564, #72836, #61103, #45811, #39077, #53454, #52121, #19677, #80049, #79609, #46707, #18352, #80957, #88169, #73295, #26444, #66540, #53906, #81395, #47141, #59774, #34959, #35405, #7940, #54787, #62420, #28198, #55669, #14696, #83615, #8386, #35858, #82277, #20562, #20994, #83161, #21894, #7502, #48920, #61988, #42617, #55232, #68309, #69633, #62859, #735, #7050, #21451, #1174, #28657, #48026, #76394, #42180, #56125, #49368, #76847, #63320, #26883, #75504, #13805, #48467, #15144, #70079, #54340, #81834, #294, #20126, #47590, #75075, #13362, #40843, #6610, #34077, #61541 ),
 ( #89046, #27325, #75954, #41290, #68752, #34523, #27761, #82721, #14251, #41731, #69195, #43496, #9704, #77278, #2063, #3389, #30425, #16468, #16910, #70970, #65081, #29546, #84058, #56568, #85375, #2495, #36305, #71399, #22770, #29986, #30858, #50231, #63759, #77719, #9277, #43934, #37174, #44360, #64635, #57001, #57889, #2939, #64190, #50679, #1630, #70527, #16027, #84494, #29111, #23661, #78165, #37622, #22337, #49801, #51113, #84939, #10158, #78605, #15587, #43052, #8834, #57443, #23219, #36738, #71848, #22812, #23694, #86318, #79549, #63799, #43529, #50270, #17396, #51146, #77759, #2098, #58815, #2531, #84973, #16948, #8871, #65568, #29585, #24591, #3427, #16065, #71887, #65120, #84535, #30894, #43970, #52056, #51592, #79093, #44851, #10197, #72330, #78649, #71006, #10641, #17847, #9315, #36774, #44398, #45299, #16503, #64230, #37658, #71438, #38105, #30024, #3867, #36340, #57041, #57484, #23254, #31353, #58361, #50716, #78203, #9744, #37211, #64676, #2978, #30458, #57929, #85413, #85856, #24140, #27588, #66918, #59264, #121, #55060, #6871, #20395, #21267, #47857, #7326, #73688, #52501, #38558, #75341, #31806, #86768, #62251, #46202, #18286, #34784, #34340, #5214, #32680, #61808, #82553, #54604, #25488, #60148, #25038, #20830, #87650, #48296 ) ),
 .UNSPECIFIED., .T., .F., .F. ) 
 B_SPLINE_SURFACE_WITH_KNOTS ( ( 4, 3, 4 ),
 ( 3, 2, 2, 2, 2, 2, 2, 2, 2, 2, 2, 2, 2, 2, 2, 2, 2, 2, 2, 2, 2, 2, 2, 2, 2, 2, 2, 2, 2, 2, 2, 2, 2, 2, 2, 2, 2, 2, 2, 2, 2, 2, 2, 2, 2, 2, 2, 2, 2, 2, 2, 2, 2, 2, 2, 2, 2, 2, 2, 2, 2, 2, 2, 2, 2, 2, 2, 2, 2, 2, 2, 2, 2, 2, 2, 2, 2, 2, 2, 2, 3 ),
 ( 0.000000000000000000, 0.5000000000000000000, 1.000000000000000000 ),
 ( 0.000000000000000000, 0.01250000000000000069, 0.02500000000000000139, 0.03749999999999999861, 0.05000000000000000278, 0.06250000000000000000, 0.07499999999999999722, 0.08749999999999999445, 0.1000000000000000056, 0.1125000000000000028, 0.1250000000000000000, 0.1375000000000000111, 0.1499999999999999944, 0.1625000000000000056, 0.1749999999999999889, 0.1875000000000000000, 0.2000000000000000111, 0.2124999999999999944, 0.2250000000000000056, 0.2374999999999999889, 0.2500000000000000000, 0.2625000000000000111, 0.2750000000000000222, 0.2874999999999999778, 0.2999999999999999889, 0.3125000000000000000, 0.3250000000000000111, 0.3375000000000000222, 0.3499999999999999778, 0.3624999999999999889, 0.3750000000000000000, 0.3875000000000000111, 0.4000000000000000222, 0.4124999999999999778, 0.4249999999999999889, 0.4375000000000000000, 0.4500000000000000111, 0.4625000000000000222, 0.4749999999999999778, 0.4874999999999999889, 0.5000000000000000000, 0.5124999999999999556, 0.5250000000000000222, 0.5374999999999999778, 0.5500000000000000444, 0.5625000000000000000, 0.5749999999999999556, 0.5875000000000000222, 0.5999999999999999778, 0.6125000000000000444, 0.6250000000000000000, 0.6374999999999999556, 0.6500000000000000222, 0.6624999999999999778, 0.6750000000000000444, 0.6875000000000000000, 0.6999999999999999556, 0.7125000000000000222, 0.7249999999999999778, 0.7375000000000000444, 0.7500000000000000000, 0.7624999999999999556, 0.7750000000000000222, 0.7874999999999999778, 0.8000000000000000444, 0.8125000000000000000, 0.8249999999999999556, 0.8375000000000000222, 0.8499999999999999778, 0.8625000000000000444, 0.8750000000000000000, 0.8874999999999999556, 0.9000000000000000222, 0.9124999999999999778, 0.9250000000000000444, 0.9375000000000000000, 0.9499999999999999556, 0.9625000000000000222, 0.9749999999999999778, 0.9875000000000000444, 1.000000000000000000 ),
 .UNSPECIFIED. ) 
 GEOMETRIC_REPRESENTATION_ITEM ( )  RATIONAL_B_SPLINE_SURFACE ( (
 ( 1.000000000000000000, 0.9238795325112867385, 1.000000000000000000, 0.9238795325112867385, 1.000000000000000000, 0.9238795325112867385, 1.000000000000000000, 0.9238795325112867385, 1.000000000000000000, 0.9238795325112867385, 1.000000000000000000, 0.9238795325112867385, 1.000000000000000000, 0.9238795325112867385, 1.000000000000000000, 0.9238795325112867385, 1.000000000000000000, 0.9238795325112867385, 1.000000000000000000, 0.9238795325112867385, 1.000000000000000000, 0.9238795325112867385, 1.000000000000000000, 0.9238795325112867385, 1.000000000000000000, 0.9238795325112867385, 1.000000000000000000, 0.9238795325112867385, 1.000000000000000000, 0.9238795325112867385, 1.000000000000000000, 0.9238795325112867385, 1.000000000000000000, 0.9238795325112867385, 1.000000000000000000, 0.9238795325112867385, 1.000000000000000000, 0.9238795325112867385, 1.000000000000000000, 0.9238795325112867385, 1.000000000000000000, 0.9238795325112867385, 1.000000000000000000, 0.9238795325112867385, 1.000000000000000000, 0.9238795325112867385, 1.000000000000000000, 0.9238795325112867385, 1.000000000000000000, 0.9238795325112867385, 1.000000000000000000, 0.9238795325112867385, 1.000000000000000000, 0.9238795325112867385, 1.000000000000000000, 0.9238795325112867385, 1.000000000000000000, 0.9238795325112867385, 1.000000000000000000, 0.9238795325112867385, 1.000000000000000000, 0.9238795325112867385, 1.000000000000000000, 0.9238795325112867385, 1.000000000000000000, 0.9238795325112867385, 1.000000000000000000, 0.9238795325112867385, 1.000000000000000000, 0.9238795325112867385, 1.000000000000000000, 0.9238795325112867385, 1.000000000000000000, 0.9238795325112867385, 1.000000000000000000, 0.9238795325112867385, 1.000000000000000000, 0.9238795325112867385, 1.000000000000000000, 0.9238795325112867385, 1.000000000000000000, 0.9238795325112867385, 1.000000000000000000, 0.9238795325112867385, 1.000000000000000000, 0.9238795325112867385, 1.000000000000000000, 0.9238795325112867385, 1.000000000000000000, 0.9238795325112867385, 1.000000000000000000, 0.9238795325112867385, 1.000000000000000000, 0.9238795325112867385, 1.000000000000000000, 0.9238795325112867385, 1.000000000000000000, 0.9238795325112867385, 1.000000000000000000, 0.9238795325112867385, 1.000000000000000000, 0.9238795325112867385, 1.000000000000000000, 0.9238795325112867385, 1.000000000000000000, 0.9238795325112867385, 1.000000000000000000, 0.9238795325112867385, 1.000000000000000000, 0.9238795325112867385, 1.000000000000000000, 0.9238795325112867385, 1.000000000000000000, 0.9238795325112867385, 1.000000000000000000, 0.9238795325112867385, 1.000000000000000000, 0.9238795325112867385, 1.000000000000000000, 0.9238795325112867385, 1.000000000000000000, 0.9238795325112867385, 1.000000000000000000, 0.9238795325112867385, 1.000000000000000000, 0.9238795325112867385, 1.000000000000000000, 0.9238795325112867385, 1.000000000000000000, 0.9238795325112867385, 1.000000000000000000, 0.9238795325112867385, 1.000000000000000000, 0.9238795325112867385, 1.000000000000000000, 0.9238795325112867385, 1.000000000000000000, 0.9238795325112867385, 1.000000000000000000, 0.9238795325112867385, 1.000000000000000000, 0.9238795325112867385, 1.000000000000000000, 0.9238795325112867385, 1.000000000000000000, 0.9238795325112867385, 1.000000000000000000, 0.9238795325112867385, 1.000000000000000000, 0.9238795325112867385, 1.000000000000000000, 0.9238795325112867385, 1.000000000000000000, 0.9238795325112867385, 1.000000000000000000, 0.9238795325112867385, 1.000000000000000000, 0.9238795325112867385, 1.000000000000000000, 0.9238795325112867385, 1.000000000000000000),
 ( 0.3333333333333333703, 0.3079598441704289313, 0.3333333333333333703, 0.3079598441704289313, 0.3333333333333333703, 0.3079598441704289313, 0.3333333333333333703, 0.3079598441704289313, 0.3333333333333333703, 0.3079598441704289313, 0.3333333333333333703, 0.3079598441704289313, 0.3333333333333333703, 0.3079598441704289313, 0.3333333333333333703, 0.3079598441704289313, 0.3333333333333333703, 0.3079598441704289313, 0.3333333333333333703, 0.3079598441704289313, 0.3333333333333333703, 0.3079598441704289313, 0.3333333333333333703, 0.3079598441704289313, 0.3333333333333333703, 0.3079598441704289313, 0.3333333333333333703, 0.3079598441704289313, 0.3333333333333333703, 0.3079598441704289313, 0.3333333333333333703, 0.3079598441704289313, 0.3333333333333333703, 0.3079598441704289313, 0.3333333333333333703, 0.3079598441704289313, 0.3333333333333333703, 0.3079598441704289313, 0.3333333333333333703, 0.3079598441704289313, 0.3333333333333333703, 0.3079598441704289313, 0.3333333333333333703, 0.3079598441704289313, 0.3333333333333333703, 0.3079598441704289313, 0.3333333333333333703, 0.3079598441704289313, 0.3333333333333333703, 0.3079598441704289313, 0.3333333333333333703, 0.3079598441704289313, 0.3333333333333333703, 0.3079598441704289313, 0.3333333333333333703, 0.3079598441704289313, 0.3333333333333333703, 0.3079598441704289313, 0.3333333333333333703, 0.3079598441704289313, 0.3333333333333333703, 0.3079598441704289313, 0.3333333333333333703, 0.3079598441704289313, 0.3333333333333333703, 0.3079598441704289313, 0.3333333333333333703, 0.3079598441704289313, 0.3333333333333333703, 0.3079598441704289313, 0.3333333333333333703, 0.3079598441704289313, 0.3333333333333333703, 0.3079598441704289313, 0.3333333333333333703, 0.3079598441704289313, 0.3333333333333333703, 0.3079598441704289313, 0.3333333333333333703, 0.3079598441704289313, 0.3333333333333333703, 0.3079598441704289313, 0.3333333333333333703, 0.3079598441704289313, 0.3333333333333333703, 0.3079598441704289313, 0.3333333333333333703, 0.3079598441704289313, 0.3333333333333333703, 0.3079598441704289313, 0.3333333333333333703, 0.3079598441704289313, 0.3333333333333333703, 0.3079598441704289313, 0.3333333333333333703, 0.3079598441704289313, 0.3333333333333333703, 0.3079598441704289313, 0.3333333333333333703, 0.3079598441704289313, 0.3333333333333333703, 0.3079598441704289313, 0.3333333333333333703, 0.3079598441704289313, 0.3333333333333333703, 0.3079598441704289313, 0.3333333333333333703, 0.3079598441704289313, 0.3333333333333333703, 0.3079598441704289313, 0.3333333333333333703, 0.3079598441704289313, 0.3333333333333333703, 0.3079598441704289313, 0.3333333333333333703, 0.3079598441704289313, 0.3333333333333333703, 0.3079598441704289313, 0.3333333333333333703, 0.3079598441704289313, 0.3333333333333333703, 0.3079598441704289313, 0.3333333333333333703, 0.3079598441704289313, 0.3333333333333333703, 0.3079598441704289313, 0.3333333333333333703, 0.3079598441704289313, 0.3333333333333333703, 0.3079598441704289313, 0.3333333333333333703, 0.3079598441704289313, 0.3333333333333333703, 0.3079598441704289313, 0.3333333333333333703, 0.3079598441704289313, 0.3333333333333333703, 0.3079598441704289313, 0.3333333333333333703, 0.3079598441704289313, 0.3333333333333333703, 0.3079598441704289313, 0.3333333333333333703, 0.3079598441704289313, 0.3333333333333333703, 0.3079598441704289313, 0.3333333333333333703, 0.3079598441704289313, 0.3333333333333333703, 0.3079598441704289313, 0.3333333333333333703, 0.3079598441704289313, 0.3333333333333333703, 0.3079598441704289313, 0.3333333333333333703, 0.3079598441704289313, 0.3333333333333333703, 0.3079598441704289313, 0.3333333333333333703, 0.3079598441704289313, 0.3333333333333333703),
 ( 0.3333333333333333703, 0.3079598441704289313, 0.3333333333333333703, 0.3079598441704289313, 0.3333333333333333703, 0.3079598441704289313, 0.3333333333333333703, 0.3079598441704289313, 0.3333333333333333703, 0.3079598441704289313, 0.3333333333333333703, 0.3079598441704289313, 0.3333333333333333703, 0.3079598441704289313, 0.3333333333333333703, 0.3079598441704289313, 0.3333333333333333703, 0.3079598441704289313, 0.3333333333333333703, 0.3079598441704289313, 0.3333333333333333703, 0.3079598441704289313, 0.3333333333333333703, 0.3079598441704289313, 0.3333333333333333703, 0.3079598441704289313, 0.3333333333333333703, 0.3079598441704289313, 0.3333333333333333703, 0.3079598441704289313, 0.3333333333333333703, 0.3079598441704289313, 0.3333333333333333703, 0.3079598441704289313, 0.3333333333333333703, 0.3079598441704289313, 0.3333333333333333703, 0.3079598441704289313, 0.3333333333333333703, 0.3079598441704289313, 0.3333333333333333703, 0.3079598441704289313, 0.3333333333333333703, 0.3079598441704289313, 0.3333333333333333703, 0.3079598441704289313, 0.3333333333333333703, 0.3079598441704289313, 0.3333333333333333703, 0.3079598441704289313, 0.3333333333333333703, 0.3079598441704289313, 0.3333333333333333703, 0.3079598441704289313, 0.3333333333333333703, 0.3079598441704289313, 0.3333333333333333703, 0.3079598441704289313, 0.3333333333333333703, 0.3079598441704289313, 0.3333333333333333703, 0.3079598441704289313, 0.3333333333333333703, 0.3079598441704289313, 0.3333333333333333703, 0.3079598441704289313, 0.3333333333333333703, 0.3079598441704289313, 0.3333333333333333703, 0.3079598441704289313, 0.3333333333333333703, 0.3079598441704289313, 0.3333333333333333703, 0.3079598441704289313, 0.3333333333333333703, 0.3079598441704289313, 0.3333333333333333703, 0.3079598441704289313, 0.3333333333333333703, 0.3079598441704289313, 0.3333333333333333703, 0.3079598441704289313, 0.3333333333333333703, 0.3079598441704289313, 0.3333333333333333703, 0.3079598441704289313, 0.3333333333333333703, 0.3079598441704289313, 0.3333333333333333703, 0.3079598441704289313, 0.3333333333333333703, 0.3079598441704289313, 0.3333333333333333703, 0.3079598441704289313, 0.3333333333333333703, 0.3079598441704289313, 0.3333333333333333703, 0.3079598441704289313, 0.3333333333333333703, 0.3079598441704289313, 0.3333333333333333703, 0.3079598441704289313, 0.3333333333333333703, 0.3079598441704289313, 0.3333333333333333703, 0.3079598441704289313, 0.3333333333333333703, 0.3079598441704289313, 0.3333333333333333703, 0.3079598441704289313, 0.3333333333333333703, 0.3079598441704289313, 0.3333333333333333703, 0.3079598441704289313, 0.3333333333333333703, 0.3079598441704289313, 0.3333333333333333703, 0.3079598441704289313, 0.3333333333333333703, 0.3079598441704289313, 0.3333333333333333703, 0.3079598441704289313, 0.3333333333333333703, 0.3079598441704289313, 0.3333333333333333703, 0.3079598441704289313, 0.3333333333333333703, 0.3079598441704289313, 0.3333333333333333703, 0.3079598441704289313, 0.3333333333333333703, 0.3079598441704289313, 0.3333333333333333703, 0.3079598441704289313, 0.3333333333333333703, 0.3079598441704289313, 0.3333333333333333703, 0.3079598441704289313, 0.3333333333333333703, 0.3079598441704289313, 0.3333333333333333703, 0.3079598441704289313, 0.3333333333333333703, 0.3079598441704289313, 0.3333333333333333703, 0.3079598441704289313, 0.3333333333333333703, 0.3079598441704289313, 0.3333333333333333703, 0.3079598441704289313, 0.3333333333333333703, 0.3079598441704289313, 0.3333333333333333703, 0.3079598441704289313, 0.3333333333333333703, 0.3079598441704289313, 0.3333333333333333703, 0.3079598441704289313, 0.3333333333333333703, 0.3079598441704289313, 0.3333333333333333703),
 ( 1.000000000000000000, 0.9238795325112867385, 1.000000000000000000, 0.9238795325112867385, 1.000000000000000000, 0.9238795325112867385, 1.000000000000000000, 0.9238795325112867385, 1.000000000000000000, 0.9238795325112867385, 1.000000000000000000, 0.9238795325112867385, 1.000000000000000000, 0.9238795325112867385, 1.000000000000000000, 0.9238795325112867385, 1.000000000000000000, 0.9238795325112867385, 1.000000000000000000, 0.9238795325112867385, 1.000000000000000000, 0.9238795325112867385, 1.000000000000000000, 0.9238795325112867385, 1.000000000000000000, 0.9238795325112867385, 1.000000000000000000, 0.9238795325112867385, 1.000000000000000000, 0.9238795325112867385, 1.000000000000000000, 0.9238795325112867385, 1.000000000000000000, 0.9238795325112867385, 1.000000000000000000, 0.9238795325112867385, 1.000000000000000000, 0.9238795325112867385, 1.000000000000000000, 0.9238795325112867385, 1.000000000000000000, 0.9238795325112867385, 1.000000000000000000, 0.9238795325112867385, 1.000000000000000000, 0.9238795325112867385, 1.000000000000000000, 0.9238795325112867385, 1.000000000000000000, 0.9238795325112867385, 1.000000000000000000, 0.9238795325112867385, 1.000000000000000000, 0.9238795325112867385, 1.000000000000000000, 0.9238795325112867385, 1.000000000000000000, 0.9238795325112867385, 1.000000000000000000, 0.9238795325112867385, 1.000000000000000000, 0.9238795325112867385, 1.000000000000000000, 0.9238795325112867385, 1.000000000000000000, 0.9238795325112867385, 1.000000000000000000, 0.9238795325112867385, 1.000000000000000000, 0.9238795325112867385, 1.000000000000000000, 0.9238795325112867385, 1.000000000000000000, 0.9238795325112867385, 1.000000000000000000, 0.9238795325112867385, 1.000000000000000000, 0.9238795325112867385, 1.000000000000000000, 0.9238795325112867385, 1.000000000000000000, 0.9238795325112867385, 1.000000000000000000, 0.9238795325112867385, 1.000000000000000000, 0.9238795325112867385, 1.000000000000000000, 0.9238795325112867385, 1.000000000000000000, 0.9238795325112867385, 1.000000000000000000, 0.9238795325112867385, 1.000000000000000000, 0.9238795325112867385, 1.000000000000000000, 0.9238795325112867385, 1.000000000000000000, 0.9238795325112867385, 1.000000000000000000, 0.9238795325112867385, 1.000000000000000000, 0.9238795325112867385, 1.000000000000000000, 0.9238795325112867385, 1.000000000000000000, 0.9238795325112867385, 1.000000000000000000, 0.9238795325112867385, 1.000000000000000000, 0.9238795325112867385, 1.000000000000000000, 0.9238795325112867385, 1.000000000000000000, 0.9238795325112867385, 1.000000000000000000, 0.9238795325112867385, 1.000000000000000000, 0.9238795325112867385, 1.000000000000000000, 0.9238795325112867385, 1.000000000000000000, 0.9238795325112867385, 1.000000000000000000, 0.9238795325112867385, 1.000000000000000000, 0.9238795325112867385, 1.000000000000000000, 0.9238795325112867385, 1.000000000000000000, 0.9238795325112867385, 1.000000000000000000, 0.9238795325112867385, 1.000000000000000000, 0.9238795325112867385, 1.000000000000000000, 0.9238795325112867385, 1.000000000000000000, 0.9238795325112867385, 1.000000000000000000, 0.9238795325112867385, 1.000000000000000000, 0.9238795325112867385, 1.000000000000000000, 0.9238795325112867385, 1.000000000000000000, 0.9238795325112867385, 1.000000000000000000, 0.9238795325112867385, 1.000000000000000000, 0.9238795325112867385, 1.000000000000000000, 0.9238795325112867385, 1.000000000000000000, 0.9238795325112867385, 1.000000000000000000, 0.9238795325112867385, 1.000000000000000000, 0.9238795325112867385, 1.000000000000000000, 0.9238795325112867385, 1.000000000000000000),
 ( 0.3333333333333333703, 0.3079598441704289313, 0.3333333333333333703, 0.3079598441704289313, 0.3333333333333333703, 0.3079598441704289313, 0.3333333333333333703, 0.3079598441704289313, 0.3333333333333333703, 0.3079598441704289313, 0.3333333333333333703, 0.3079598441704289313, 0.3333333333333333703, 0.3079598441704289313, 0.3333333333333333703, 0.3079598441704289313, 0.3333333333333333703, 0.3079598441704289313, 0.3333333333333333703, 0.3079598441704289313, 0.3333333333333333703, 0.3079598441704289313, 0.3333333333333333703, 0.3079598441704289313, 0.3333333333333333703, 0.3079598441704289313, 0.3333333333333333703, 0.3079598441704289313, 0.3333333333333333703, 0.3079598441704289313, 0.3333333333333333703, 0.3079598441704289313, 0.3333333333333333703, 0.3079598441704289313, 0.3333333333333333703, 0.3079598441704289313, 0.3333333333333333703, 0.3079598441704289313, 0.3333333333333333703, 0.3079598441704289313, 0.3333333333333333703, 0.3079598441704289313, 0.3333333333333333703, 0.3079598441704289313, 0.3333333333333333703, 0.3079598441704289313, 0.3333333333333333703, 0.3079598441704289313, 0.3333333333333333703, 0.3079598441704289313, 0.3333333333333333703, 0.3079598441704289313, 0.3333333333333333703, 0.3079598441704289313, 0.3333333333333333703, 0.3079598441704289313, 0.3333333333333333703, 0.3079598441704289313, 0.3333333333333333703, 0.3079598441704289313, 0.3333333333333333703, 0.3079598441704289313, 0.3333333333333333703, 0.3079598441704289313, 0.3333333333333333703, 0.3079598441704289313, 0.3333333333333333703, 0.3079598441704289313, 0.3333333333333333703, 0.3079598441704289313, 0.3333333333333333703, 0.3079598441704289313, 0.3333333333333333703, 0.3079598441704289313, 0.3333333333333333703, 0.3079598441704289313, 0.3333333333333333703, 0.3079598441704289313, 0.3333333333333333703, 0.3079598441704289313, 0.3333333333333333703, 0.3079598441704289313, 0.3333333333333333703, 0.3079598441704289313, 0.3333333333333333703, 0.3079598441704289313, 0.3333333333333333703, 0.3079598441704289313, 0.3333333333333333703, 0.3079598441704289313, 0.3333333333333333703, 0.3079598441704289313, 0.3333333333333333703, 0.3079598441704289313, 0.3333333333333333703, 0.3079598441704289313, 0.3333333333333333703, 0.3079598441704289313, 0.3333333333333333703, 0.3079598441704289313, 0.3333333333333333703, 0.3079598441704289313, 0.3333333333333333703, 0.3079598441704289313, 0.3333333333333333703, 0.3079598441704289313, 0.3333333333333333703, 0.3079598441704289313, 0.3333333333333333703, 0.3079598441704289313, 0.3333333333333333703, 0.3079598441704289313, 0.3333333333333333703, 0.3079598441704289313, 0.3333333333333333703, 0.3079598441704289313, 0.3333333333333333703, 0.3079598441704289313, 0.3333333333333333703, 0.3079598441704289313, 0.3333333333333333703, 0.3079598441704289313, 0.3333333333333333703, 0.3079598441704289313, 0.3333333333333333703, 0.3079598441704289313, 0.3333333333333333703, 0.3079598441704289313, 0.3333333333333333703, 0.3079598441704289313, 0.3333333333333333703, 0.3079598441704289313, 0.3333333333333333703, 0.3079598441704289313, 0.3333333333333333703, 0.3079598441704289313, 0.3333333333333333703, 0.3079598441704289313, 0.3333333333333333703, 0.3079598441704289313, 0.3333333333333333703, 0.3079598441704289313, 0.3333333333333333703, 0.3079598441704289313, 0.3333333333333333703, 0.3079598441704289313, 0.3333333333333333703, 0.3079598441704289313, 0.3333333333333333703, 0.3079598441704289313, 0.3333333333333333703, 0.3079598441704289313, 0.3333333333333333703, 0.3079598441704289313, 0.3333333333333333703, 0.3079598441704289313, 0.3333333333333333703, 0.3079598441704289313, 0.3333333333333333703, 0.3079598441704289313, 0.3333333333333333703),
 ( 0.3333333333333333703, 0.3079598441704289313, 0.3333333333333333703, 0.3079598441704289313, 0.3333333333333333703, 0.3079598441704289313, 0.3333333333333333703, 0.3079598441704289313, 0.3333333333333333703, 0.3079598441704289313, 0.3333333333333333703, 0.3079598441704289313, 0.3333333333333333703, 0.3079598441704289313, 0.3333333333333333703, 0.3079598441704289313, 0.3333333333333333703, 0.3079598441704289313, 0.3333333333333333703, 0.3079598441704289313, 0.3333333333333333703, 0.3079598441704289313, 0.3333333333333333703, 0.3079598441704289313, 0.3333333333333333703, 0.3079598441704289313, 0.3333333333333333703, 0.3079598441704289313, 0.3333333333333333703, 0.3079598441704289313, 0.3333333333333333703, 0.3079598441704289313, 0.3333333333333333703, 0.3079598441704289313, 0.3333333333333333703, 0.3079598441704289313, 0.3333333333333333703, 0.3079598441704289313, 0.3333333333333333703, 0.3079598441704289313, 0.3333333333333333703, 0.3079598441704289313, 0.3333333333333333703, 0.3079598441704289313, 0.3333333333333333703, 0.3079598441704289313, 0.3333333333333333703, 0.3079598441704289313, 0.3333333333333333703, 0.3079598441704289313, 0.3333333333333333703, 0.3079598441704289313, 0.3333333333333333703, 0.3079598441704289313, 0.3333333333333333703, 0.3079598441704289313, 0.3333333333333333703, 0.3079598441704289313, 0.3333333333333333703, 0.3079598441704289313, 0.3333333333333333703, 0.3079598441704289313, 0.3333333333333333703, 0.3079598441704289313, 0.3333333333333333703, 0.3079598441704289313, 0.3333333333333333703, 0.3079598441704289313, 0.3333333333333333703, 0.3079598441704289313, 0.3333333333333333703, 0.3079598441704289313, 0.3333333333333333703, 0.3079598441704289313, 0.3333333333333333703, 0.3079598441704289313, 0.3333333333333333703, 0.3079598441704289313, 0.3333333333333333703, 0.3079598441704289313, 0.3333333333333333703, 0.3079598441704289313, 0.3333333333333333703, 0.3079598441704289313, 0.3333333333333333703, 0.3079598441704289313, 0.3333333333333333703, 0.3079598441704289313, 0.3333333333333333703, 0.3079598441704289313, 0.3333333333333333703, 0.3079598441704289313, 0.3333333333333333703, 0.3079598441704289313, 0.3333333333333333703, 0.3079598441704289313, 0.3333333333333333703, 0.3079598441704289313, 0.3333333333333333703, 0.3079598441704289313, 0.3333333333333333703, 0.3079598441704289313, 0.3333333333333333703, 0.3079598441704289313, 0.3333333333333333703, 0.3079598441704289313, 0.3333333333333333703, 0.3079598441704289313, 0.3333333333333333703, 0.3079598441704289313, 0.3333333333333333703, 0.3079598441704289313, 0.3333333333333333703, 0.3079598441704289313, 0.3333333333333333703, 0.3079598441704289313, 0.3333333333333333703, 0.3079598441704289313, 0.3333333333333333703, 0.3079598441704289313, 0.3333333333333333703, 0.3079598441704289313, 0.3333333333333333703, 0.3079598441704289313, 0.3333333333333333703, 0.3079598441704289313, 0.3333333333333333703, 0.3079598441704289313, 0.3333333333333333703, 0.3079598441704289313, 0.3333333333333333703, 0.3079598441704289313, 0.3333333333333333703, 0.3079598441704289313, 0.3333333333333333703, 0.3079598441704289313, 0.3333333333333333703, 0.3079598441704289313, 0.3333333333333333703, 0.3079598441704289313, 0.3333333333333333703, 0.3079598441704289313, 0.3333333333333333703, 0.3079598441704289313, 0.3333333333333333703, 0.3079598441704289313, 0.3333333333333333703, 0.3079598441704289313, 0.3333333333333333703, 0.3079598441704289313, 0.3333333333333333703, 0.3079598441704289313, 0.3333333333333333703, 0.3079598441704289313, 0.3333333333333333703, 0.3079598441704289313, 0.3333333333333333703, 0.3079598441704289313, 0.3333333333333333703, 0.3079598441704289313, 0.3333333333333333703),
 ( 1.000000000000000000, 0.9238795325112867385, 1.000000000000000000, 0.9238795325112867385, 1.000000000000000000, 0.9238795325112867385, 1.000000000000000000, 0.9238795325112867385, 1.000000000000000000, 0.9238795325112867385, 1.000000000000000000, 0.9238795325112867385, 1.000000000000000000, 0.9238795325112867385, 1.000000000000000000, 0.9238795325112867385, 1.000000000000000000, 0.9238795325112867385, 1.000000000000000000, 0.9238795325112867385, 1.000000000000000000, 0.9238795325112867385, 1.000000000000000000, 0.9238795325112867385, 1.000000000000000000, 0.9238795325112867385, 1.000000000000000000, 0.9238795325112867385, 1.000000000000000000, 0.9238795325112867385, 1.000000000000000000, 0.9238795325112867385, 1.000000000000000000, 0.9238795325112867385, 1.000000000000000000, 0.9238795325112867385, 1.000000000000000000, 0.9238795325112867385, 1.000000000000000000, 0.9238795325112867385, 1.000000000000000000, 0.9238795325112867385, 1.000000000000000000, 0.9238795325112867385, 1.000000000000000000, 0.9238795325112867385, 1.000000000000000000, 0.9238795325112867385, 1.000000000000000000, 0.9238795325112867385, 1.000000000000000000, 0.9238795325112867385, 1.000000000000000000, 0.9238795325112867385, 1.000000000000000000, 0.9238795325112867385, 1.000000000000000000, 0.9238795325112867385, 1.000000000000000000, 0.9238795325112867385, 1.000000000000000000, 0.9238795325112867385, 1.000000000000000000, 0.9238795325112867385, 1.000000000000000000, 0.9238795325112867385, 1.000000000000000000, 0.9238795325112867385, 1.000000000000000000, 0.9238795325112867385, 1.000000000000000000, 0.9238795325112867385, 1.000000000000000000, 0.9238795325112867385, 1.000000000000000000, 0.9238795325112867385, 1.000000000000000000, 0.9238795325112867385, 1.000000000000000000, 0.9238795325112867385, 1.000000000000000000, 0.9238795325112867385, 1.000000000000000000, 0.9238795325112867385, 1.000000000000000000, 0.9238795325112867385, 1.000000000000000000, 0.9238795325112867385, 1.000000000000000000, 0.9238795325112867385, 1.000000000000000000, 0.9238795325112867385, 1.000000000000000000, 0.9238795325112867385, 1.000000000000000000, 0.9238795325112867385, 1.000000000000000000, 0.9238795325112867385, 1.000000000000000000, 0.9238795325112867385, 1.000000000000000000, 0.9238795325112867385, 1.000000000000000000, 0.9238795325112867385, 1.000000000000000000, 0.9238795325112867385, 1.000000000000000000, 0.9238795325112867385, 1.000000000000000000, 0.9238795325112867385, 1.000000000000000000, 0.9238795325112867385, 1.000000000000000000, 0.9238795325112867385, 1.000000000000000000, 0.9238795325112867385, 1.000000000000000000, 0.9238795325112867385, 1.000000000000000000, 0.9238795325112867385, 1.000000000000000000, 0.9238795325112867385, 1.000000000000000000, 0.9238795325112867385, 1.000000000000000000, 0.9238795325112867385, 1.000000000000000000, 0.9238795325112867385, 1.000000000000000000, 0.9238795325112867385, 1.000000000000000000, 0.9238795325112867385, 1.000000000000000000, 0.9238795325112867385, 1.000000000000000000, 0.9238795325112867385, 1.000000000000000000, 0.9238795325112867385, 1.000000000000000000, 0.9238795325112867385, 1.000000000000000000, 0.9238795325112867385, 1.000000000000000000, 0.9238795325112867385, 1.000000000000000000, 0.9238795325112867385, 1.000000000000000000, 0.9238795325112867385, 1.000000000000000000, 0.9238795325112867385, 1.000000000000000000, 0.9238795325112867385, 1.000000000000000000, 0.9238795325112867385, 1.000000000000000000, 0.9238795325112867385, 1.000000000000000000, 0.9238795325112867385, 1.000000000000000000, 0.9238795325112867385, 1.000000000000000000) ) ) 
 REPRESENTATION_ITEM ( '' )  SURFACE ( )  );
#35807=CARTESIAN_POINT ( 'NONE',  ( -3.750000000000007550, -5.946699141100917352, 26.42187500000000000 ) ) ;
#35836=CARTESIAN_POINT ( 'NONE',  ( -1.901340078031346525, -9.487747218494661183, 24.68563170625849068 ) ) ;
#35838=CARTESIAN_POINT ( 'NONE',  ( -2.333004543783647744, -4.556662903998644154, 13.99999999999999289 ) ) ;
#35846=CARTESIAN_POINT ( 'NONE',  ( 1.200186371490561621, -10.22469193450123193, 23.20125670625849068 ) ) ;
#35854=CARTESIAN_POINT ( 'NONE',  ( -3.749999999999988454, -9.053300858899127945, 17.51562500000000000 ) ) ;
#35858=CARTESIAN_POINT ( 'NONE',  ( 3.750000000000001776, -7.561099074964511502, 22.22061829374151287 ) ) ;
#35943=CARTESIAN_POINT ( 'NONE',  ( 1.492201783934554493, -3.724691934501233703, 18.98250670625849068 ) ) ;
#35951=CARTESIAN_POINT ( 'NONE',  ( 1.614399933863660985, -11.22469193450123193, 23.20125670625849068 ) ) ;
#35966=CARTESIAN_POINT ( 'NONE',  ( -1.987747218494638313, -9.401340078031370950, 21.43936829374151642 ) ) ;
#35975=CARTESIAN_POINT ( 'NONE',  ( -2.749999999999998224, -7.500000000000015987, 26.34375000000000000 ) ) ;
#36051=CARTESIAN_POINT ( 'NONE',  ( -1.553300858899125059, -3.750000000000009326, 16.57812500000000000 ) ) ;
#36075=CARTESIAN_POINT ( 'NONE',  ( -2.608446859217920633, -4.805146000318815780, 14.25186829374151465 ) ) ;
#36079=CARTESIAN_POINT ( 'NONE',  ( 1.944543648262996083, -5.555456351736983045, 20.56250000000000000 ) ) ;
#36186=CARTESIAN_POINT ( 'NONE',  ( -1.944543648262992530, -9.444543648263016067, 24.93750000000000000 ) ) ;
#36247=CARTESIAN_POINT ( 'NONE',  ( 2.320192649118979489E-14, -11.25000000000000000, 23.53125000000000000 ) ) ;
#36278=CIRCLE ( 'NONE', #70796, 0.4999999999999994449 ) ;
#36280=CARTESIAN_POINT ( 'NONE',  ( -1.077988221561460236, -10.27530806549876452, 23.35750670625849423 ) ) ;
#36282=CARTESIAN_POINT ( 'NONE',  ( 3.318022706343656925, -6.194818042847236583, 14.00000000000015099 ) ) ;
#36290=CARTESIAN_POINT ( 'NONE',  ( 2.750000000000001332, -7.438900925035452083, 22.96688170625849068 ) ) ;
#36298=CARTESIAN_POINT ( 'NONE',  ( -1.929879867024197893E-14, -3.750000000000000000, 14.15625000000000000 ) ) ;
#36305=CARTESIAN_POINT ( 'NONE',  ( 2.320192649118979489E-14, -11.25000000000000000, 16.03125000000000000 ) ) ;
#36340=CARTESIAN_POINT ( 'NONE',  ( -2.651650429449565305, -4.848349570550461785, 22.75000000000000000 ) ) ;
#36382=CARTESIAN_POINT ( 'NONE',  ( 1.492201783934554493, -3.724691934501233703, 21.48250670625849068 ) ) ;
#36390=CARTESIAN_POINT ( 'NONE',  ( -1.614399933863656544, -3.775308065498769405, 22.57625670625848713 ) ) ;
#36408=CARTESIAN_POINT ( 'NONE',  ( 3.775308065498752086, -6.007798216065404873, 14.64249329374151110 ) ) ;
#36487=CARTESIAN_POINT ( 'NONE',  ( -3.750000000000008438, -5.946699141100917352, 17.67187500000000355 ) ) ;
#36499=CARTESIAN_POINT ( 'NONE',  ( -1.929879867024197893E-14, -3.750000000000000000, 19.15625000000000000 ) ) ;
#36513=CARTESIAN_POINT ( 'NONE',  ( 1.077988221561497539, -10.27530806549875386, 24.95499329374151287 ) ) ;
#36518=CARTESIAN_POINT ( 'NONE',  ( -2.750000000000007105, -6.360912703474006946, 18.92187500000000355 ) ) ;
#36524=CARTESIAN_POINT ( 'NONE',  ( 1.944543648263018731, -9.444543648262994751, 14.62500000000000000 ) ) ;
#36615=CARTESIAN_POINT ( 'NONE',  ( -2.749999999999991562, -8.639087296526025028, 22.51562500000000000 ) ) ;
#36713=CARTESIAN_POINT ( 'NONE',  ( -1.901340078031346525, -9.487747218494661183, 20.93563170625849068 ) ) ;
#36715=CARTESIAN_POINT ( 'NONE',  ( 3.116851723387825235, -7.815776116252264316, 14.00000000000001066 ) ) ;
#36724=CARTESIAN_POINT ( 'NONE',  ( -1.077988221561460236, -10.27530806549876452, 23.35750670625849423 ) ) ;
#36732=CARTESIAN_POINT ( 'NONE',  ( 3.750000000000009770, -9.053300858899081760, 17.04687500000000000 ) ) ;
#36738=CARTESIAN_POINT ( 'NONE',  ( -3.750000000000008438, -5.946699141100917352, 18.92187500000000355 ) ) ;
#36774=CARTESIAN_POINT ( 'NONE',  ( 3.750000000000000888, -7.499999999999978684, 21.96875000000000355 ) ) ;
#36814=CARTESIAN_POINT ( 'NONE',  ( 1.614399933863660985, -11.22469193450123193, 19.45125670625849068 ) ) ;
#36824=CARTESIAN_POINT ( 'NONE',  ( 3.775308065498768517, -8.992201783934554271, 20.54500670625849068 ) ) ;
#36837=CARTESIAN_POINT ( 'NONE',  ( 3.724691934501251023, -9.114399933863618131, 14.79874329374151642 ) ) ;
#36913=CARTESIAN_POINT ( 'NONE',  ( 2.651650429449539104, -4.848349570550432475, 18.06250000000000355 ) ) ;
#36924=CARTESIAN_POINT ( 'NONE',  ( 3.750000000000000888, -7.499999999999978684, 19.46875000000000000 ) ) ;
#36937=CARTESIAN_POINT ( 'NONE',  ( -2.749999999999999112, -7.438900925035484057, 24.09561829374151287 ) ) ;
#36941=CARTESIAN_POINT ( 'NONE',  ( -1.077988221561493543, -4.724691934501247914, 13.07999329374151642 ) ) ;
#36946=CARTESIAN_POINT ( 'NONE',  ( -1.409462824231155764E-14, -4.749999999999999112, 14.15625000000000000 ) ) ;
#37038=CARTESIAN_POINT ( 'NONE',  ( 1.139087296526029469, -10.24999999999999467, 24.70312500000000000 ) ) ;
#37147=CARTESIAN_POINT ( 'NONE',  ( -1.987747218494660295, -5.598659921968651254, 21.24813170625848713 ) ) ;
#37160=CARTESIAN_POINT ( 'NONE',  ( 1.200186371490561621, -10.22469193450123193, 25.70125670625848713 ) ) ;
#37169=CARTESIAN_POINT ( 'NONE',  ( 1.553300858899129944, -11.24999999999998934, 15.95312500000000000 ) ) ;
#37174=CARTESIAN_POINT ( 'NONE',  ( 2.651650429449539104, -4.848349570550432475, 16.81250000000000000 ) ) ;
#37211=CARTESIAN_POINT ( 'NONE',  ( 1.553300858899129944, -11.24999999999998934, 23.45312500000000000 ) ) ;
#37246=CARTESIAN_POINT ( 'NONE',  ( -3.775308065498766297, -6.007798216065450170, 21.17000670625848713 ) ) ;
#37258=CARTESIAN_POINT ( 'NONE',  ( -1.492201783934549164, -11.27530806549876807, 19.60750670625849068 ) ) ;
#37275=CARTESIAN_POINT ( 'NONE',  ( 3.724691934501251023, -9.114399933863618131, 16.04874329374151287 ) ) ;
#37351=CARTESIAN_POINT ( 'NONE',  ( 1.553300858899087311, -3.749999999999992006, 16.73437500000000000 ) ) ;
#37362=CARTESIAN_POINT ( 'NONE',  ( -3.750000000000008438, -5.946699141100917352, 20.17187500000000000 ) ) ;
#37376=CARTESIAN_POINT ( 'NONE',  ( -3.775308065498748977, -8.992201783934593351, 20.26749329374151998 ) ) ;
#37381=CARTESIAN_POINT ( 'NONE',  ( -2.749999999999998224, -7.500000000000015987, 23.84375000000000000 ) ) ;
#37387=CARTESIAN_POINT ( 'NONE',  ( -1.944543648263014957, -5.555456351737005249, 17.75000000000000355 ) ) ;
#37432=ADVANCED_BREP_SHAPE_REPRESENTATION ( '', ( #9, #83448 ), #34517 ) ;
#37485=CARTESIAN_POINT ( 'NONE',  ( -1.901340078031369618, -5.512252781505359245, 15.50186829374151287 ) ) ;
#37517=CARTESIAN_POINT ( 'NONE',  ( -2.298097038856290464, -5.201902961143733961, 14.00000000000000000 ) ) ;
#37594=CARTESIAN_POINT ( 'NONE',  ( 1.944543648262996083, -5.555456351736983045, 14.31250000000000000 ) ) ;
#37605=CARTESIAN_POINT ( 'NONE',  ( -2.749999999999997780, -7.561099074964547917, 26.09188170625848358 ) ) ;
#37615=CARTESIAN_POINT ( 'NONE',  ( 3.750000000000009770, -9.053300858899081760, 15.79687500000000178 ) ) ;
#37622=CARTESIAN_POINT ( 'NONE',  ( 1.553300858899087311, -3.749999999999992006, 17.98437500000000000 ) ) ;
#37658=CARTESIAN_POINT ( 'NONE',  ( -1.553300858899081538, -11.25000000000000711, 22.35937500000000711 ) ) ;
#37668=CARTESIAN_POINT ( 'NONE',  ( -1.553300858899125059, -3.750000000000009326, 15.32812500000000178 ) ) ;
#37698=CARTESIAN_POINT ( 'NONE',  ( -3.724691934501229262, -9.114399933863657211, 21.01375670625849068 ) ) ;
#37708=CARTESIAN_POINT ( 'NONE',  ( 0.06109907496455496689, -11.24999999999999822, 19.52938170625848713 ) ) ;
#37723=CARTESIAN_POINT ( 'NONE',  ( 2.694853999681185108, -4.891553140782077591, 15.81436829374151465 ) ) ;
#37805=CARTESIAN_POINT ( 'NONE',  ( 2.651650429449539104, -4.848349570550432475, 19.31250000000000000 ) ) ;
#37815=CARTESIAN_POINT ( 'NONE',  ( 1.553300858899087311, -3.749999999999992006, 17.98437500000000000 ) ) ;
#37828=CARTESIAN_POINT ( 'NONE',  ( -2.608446859217920633, -4.805146000318815780, 19.25186829374151287 ) ) ;
#37833=CARTESIAN_POINT ( 'NONE',  ( 2.750000000000001776, -7.499999999999984013, 25.71875000000000000 ) ) ;
#37840=CARTESIAN_POINT ( 'NONE',  ( -1.409462824231155764E-14, -4.749999999999999112, 17.90625000000000000 ) ) ;
#37941=CARTESIAN_POINT ( 'NONE',  ( 2.750000000000002665, -7.561099074964516831, 13.47061829374151465 ) ) ;
#38048=CARTESIAN_POINT ( 'NONE',  ( -2.749999999999998224, -7.500000000000015987, 15.09375000000000000 ) ) ;
#38050=CARTESIAN_POINT ( 'NONE',  ( 3.056863809964074807, -7.383657973411067665, 13.99999999999999467 ) ) ;
#38057=CARTESIAN_POINT ( 'NONE',  ( -1.944543648262992530, -9.444543648263016067, 16.18750000000000000 ) ) ;
#38066=CARTESIAN_POINT ( 'NONE',  ( 2.651650429449569302, -10.15165042944953733, 19.62500000000000000 ) ) ;
#38105=CARTESIAN_POINT ( 'NONE',  ( -3.749999999999988454, -9.053300858899127945, 22.51562500000000000 ) ) ;
#38112=CARTESIAN_POINT ( 'NONE',  ( -1.929879867024197893E-14, -3.750000000000000000, 17.90625000000000000 ) ) ;
#38124=EDGE_CURVE ( 'NONE', #76825, #28286, #32837, .T. ) ;
#38146=CARTESIAN_POINT ( 'NONE',  ( 3.749999999999999556, -7.438900925035446754, 22.96688170625849068 ) ) ;
#38156=CARTESIAN_POINT ( 'NONE',  ( -1.987747218494660295, -5.598659921968651254, 14.99813170625848713 ) ) ;
#38169=CARTESIAN_POINT ( 'NONE',  ( 2.724691934501250135, -8.700186371490531201, 24.79874329374151998 ) ) ;
#38256=CARTESIAN_POINT ( 'NONE',  ( -3.749999999999988454, -9.053300858899127945, 22.51562500000000000 ) ) ;
#38265=CARTESIAN_POINT ( 'NONE',  ( 2.651650429449569302, -10.15165042944953733, 18.37500000000000355 ) ) ;
#38286=CARTESIAN_POINT ( 'NONE',  ( -1.409462824231155764E-14, -4.749999999999999112, 24.15625000000000000 ) ) ;
#38292=CARTESIAN_POINT ( 'NONE',  ( -2.749999999999991562, -8.639087296526026805, 18.76562500000000000 ) ) ;
#38385=CARTESIAN_POINT ( 'NONE',  ( 1.200186371490529202, -4.775308065498752974, 13.23624329374151465 ) ) ;
#38386=ORIENTED_EDGE ( 'NONE', *, *, #18440, .T. ) ;
#38497=CARTESIAN_POINT ( 'NONE',  ( -1.901340078031346525, -9.487747218494661183, 25.93563170625849423 ) ) ;
#38507=CARTESIAN_POINT ( 'NONE',  ( -2.749999999999991562, -8.639087296526025028, 16.26562500000000000 ) ) ;
#38515=CARTESIAN_POINT ( 'NONE',  ( 2.651650429449569302, -10.15165042944953733, 20.87500000000000000 ) ) ;
#38558=CARTESIAN_POINT ( 'NONE',  ( -3.749999999999988454, -9.053300858899127945, 25.01562500000000000 ) ) ;
#38596=CARTESIAN_POINT ( 'NONE',  ( 0.06109907496455496689, -11.24999999999999822, 24.52938170625849423 ) ) ;
#38606=CARTESIAN_POINT ( 'NONE',  ( 3.775308065498768517, -8.992201783934554271, 25.54500670625849779 ) ) ;
#38619=CARTESIAN_POINT ( 'NONE',  ( -1.492201783934593573, -3.724691934501250135, 18.07999329374151287 ) ) ;
#38695=DIRECTION ( 'NONE',  ( -0.7071067811865510144, 0.7071067811865440200, 0.000000000000000000 ) ) ;
#38700=CARTESIAN_POINT ( 'NONE',  ( -1.553300858899081538, -11.25000000000000711, 23.60937500000000711 ) ) ;
#38710=CARTESIAN_POINT ( 'NONE',  ( 1.553300858899129944, -11.24999999999998934, 20.95312500000000000 ) ) ;
#38729=CARTESIAN_POINT ( 'NONE',  ( 1.987747218494642309, -5.598659921968629050, 17.06436829374151287 ) ) ;
#38736=CARTESIAN_POINT ( 'NONE',  ( 1.944543648263018731, -9.444543648262994751, 19.62500000000000000 ) ) ;
#38838=CARTESIAN_POINT ( 'NONE',  ( -1.987747218494638313, -9.401340078031370950, 17.68936829374151287 ) ) ;
#38862=( NAMED_UNIT ( * ) PLANE_ANGLE_UNIT ( ) SI_UNIT ( $, .RADIAN. ) );
#38952=CARTESIAN_POINT ( 'NONE',  ( -1.987747218494660295, -5.598659921968651254, 27.49813170625849068 ) ) ;
#38962=CARTESIAN_POINT ( 'NONE',  ( 2.750000000000001332, -7.438900925035452083, 26.71688170625849068 ) ) ;
#38972=CARTESIAN_POINT ( 'NONE',  ( 1.553300858899129944, -11.24999999999998934, 23.45312500000000000 ) ) ;
#39021=CARTESIAN_POINT ( 'NONE',  ( -1.553300858899125059, -3.750000000000009326, 16.57812500000000000 ) ) ;
#39055=CARTESIAN_POINT ( 'NONE',  ( -0.06109907496455085213, -3.750000000000000888, 23.90438170625849068 ) ) ;
#39065=CARTESIAN_POINT ( 'NONE',  ( -3.749999999999996447, -7.561099074964554134, 24.84188170625848713 ) ) ;
#39077=CARTESIAN_POINT ( 'NONE',  ( -1.614399933863613468, -11.22469193450124969, 20.11124329374151642 ) ) ;
#39161=CARTESIAN_POINT ( 'NONE',  ( -3.749999999999988454, -9.053300858899127945, 23.76562499999999645 ) ) ;
#39164=( BOUNDED_CURVE ( )  B_SPLINE_CURVE ( 3, ( #87572, #19093, #53308, #88904 ),
 .UNSPECIFIED., .F., .F. ) 
 B_SPLINE_CURVE_WITH_KNOTS ( ( 4, 4 ),
 ( 1.570796326794895892, 1.579613961134529010 ),
 .UNSPECIFIED. ) 
 CURVE ( )  GEOMETRIC_REPRESENTATION_ITEM ( )  RATIONAL_B_SPLINE_CURVE ( ( 1.000000000000000000, 0.9999935207875494392, 0.9999935207875494392, 1.000000000000000000 ) ) 
 REPRESENTATION_ITEM ( '' )  );
#39171=CARTESIAN_POINT ( 'NONE',  ( -3.749999999999988454, -9.053300858899127945, 22.51562500000000000 ) ) ;
#39188=CARTESIAN_POINT ( 'NONE',  ( 2.775308065498755195, -6.422011778438505125, 18.39249329374151642 ) ) ;
#39193=CARTESIAN_POINT ( 'NONE',  ( -1.944543648262992530, -9.444543648263016067, 18.68750000000000000 ) ) ;
#39289=CARTESIAN_POINT ( 'NONE',  ( 1.901340078031373171, -9.487747218494639867, 14.87686829374151465 ) ) ;
#39398=CARTESIAN_POINT ( 'NONE',  ( -1.139087296526025916, -4.750000000000006217, 16.57812500000000000 ) ) ;
#39409=CARTESIAN_POINT ( 'NONE',  ( 1.944543648263018731, -9.444543648262994751, 15.87500000000000000 ) ) ;
#39417=CARTESIAN_POINT ( 'NONE',  ( -2.651650429449565305, -4.848349570550461785, 20.25000000000000000 ) ) ;
#39466=CARTESIAN_POINT ( 'NONE',  ( -3.750000000000007550, -5.946699141100917352, 16.42187500000000000 ) ) ;
#39498=CARTESIAN_POINT ( 'NONE',  ( -2.694853999681210865, -4.891553140782108677, 24.99813170625849423 ) ) ;
#39509=CARTESIAN_POINT ( 'NONE',  ( 2.694853999681214862, -10.10844685921789043, 25.62313170625849068 ) ) ;
#39516=CARTESIAN_POINT ( 'NONE',  ( 3.750000000000001776, -7.561099074964511502, 15.97061829374151287 ) ) ;
#39524=CARTESIAN_POINT ( 'NONE',  ( -2.608446859217920633, -4.805146000318815780, 18.00186829374151287 ) ) ;
#39610=CARTESIAN_POINT ( 'NONE',  ( 3.749999999999992006, -5.946699141100872943, 19.39062500000000711 ) ) ;
#39618=CARTESIAN_POINT ( 'NONE',  ( -1.929879867024197893E-14, -3.750000000000000000, 24.15625000000000000 ) ) ;
#39635=CARTESIAN_POINT ( 'NONE',  ( -2.775308065498752086, -8.577988221561495763, 14.01749329374151642 ) ) ;
#39641=CARTESIAN_POINT ( 'NONE',  ( 1.139087296525997051, -4.749999999999992895, 22.98437500000000000 ) ) ;
#39732=CARTESIAN_POINT ( 'NONE',  ( 2.775308065498755195, -6.422011778438505125, 20.89249329374151642 ) ) ;
#39796=CARTESIAN_POINT ( 'NONE',  ( 1.653273178848927064E-15, -7.500000000000000000, 14.00000000000000178 ) ) ;
#39835=CARTESIAN_POINT ( 'NONE',  ( -1.944543648263014957, -5.555456351737005249, 19.00000000000000000 ) ) ;
#39846=CARTESIAN_POINT ( 'NONE',  ( -1.409462824231155764E-14, -4.749999999999999112, 15.40625000000000000 ) ) ;
#39854=CARTESIAN_POINT ( 'NONE',  ( 2.651650429449539104, -4.848349570550432475, 23.06250000000000000 ) ) ;
#39908=CARTESIAN_POINT ( 'NONE',  ( 2.651650429449539104, -4.848349570550432475, 18.06250000000000355 ) ) ;
#39939=CARTESIAN_POINT ( 'NONE',  ( -0.06109907496455085213, -3.750000000000000888, 25.15438170625849068 ) ) ;
#39951=CARTESIAN_POINT ( 'NONE',  ( 0.06109907496455496689, -11.24999999999999822, 27.02938170625848358 ) ) ;
#39959=CARTESIAN_POINT ( 'NONE',  ( -1.492201783934593573, -3.724691934501250135, 16.82999329374151287 ) ) ;
#39966=CARTESIAN_POINT ( 'NONE',  ( -3.724691934501248802, -5.885600066136383646, 19.17374329374151642 ) ) ;
#40053=CARTESIAN_POINT ( 'NONE',  ( 1.553300858899129944, -11.24999999999998934, 20.95312500000000000 ) ) ;
#40062=CARTESIAN_POINT ( 'NONE',  ( -2.651650429449535551, -10.15165042944956753, 21.18750000000000000 ) ) ;
#40082=CARTESIAN_POINT ( 'NONE',  ( -2.724691934501246582, -6.299813628509474128, 16.67374329374151998 ) ) ;
#40088=CARTESIAN_POINT ( 'NONE',  ( -2.749999999999998224, -7.500000000000015987, 23.84375000000000000 ) ) ;
#40156=PRODUCT_CONTEXT ( 'NONE', #80885, 'mechanical' ) ;
#40178=CARTESIAN_POINT ( 'NONE',  ( 1.901340078031373171, -9.487747218494639867, 18.62686829374151642 ) ) ;
#40283=CARTESIAN_POINT ( 'NONE',  ( -1.944543648262992530, -9.444543648263016067, 19.93750000000000000 ) ) ;
#40291=CARTESIAN_POINT ( 'NONE',  ( 2.750000000000008438, -8.639087296525996607, 22.04687500000000000 ) ) ;
#40345=CARTESIAN_POINT ( 'NONE',  ( -2.651650429449535551, -10.15165042944956753, 19.93750000000000000 ) ) ;
#40381=CARTESIAN_POINT ( 'NONE',  ( 1.200186371490561621, -10.22469193450123193, 15.70125670625848890 ) ) ;
#40395=CARTESIAN_POINT ( 'NONE',  ( -2.749999999999997780, -7.561099074964547917, 17.34188170625849068 ) ) ;
#40403=CARTESIAN_POINT ( 'NONE',  ( 1.614399933863618797, -3.775308065498751198, 21.98624329374151642 ) ) ;
#40410=CARTESIAN_POINT ( 'NONE',  ( 3.775308065498752086, -6.007798216065404873, 17.14249329374151287 ) ) ;
#40492=CARTESIAN_POINT ( 'NONE',  ( 2.608446859217893099, -4.805146000318787358, 15.31063170625849068 ) ) ;
#40503=CARTESIAN_POINT ( 'NONE',  ( 3.749999999999992006, -5.946699141100872943, 20.64062500000000000 ) ) ;
#40518=CARTESIAN_POINT ( 'NONE',  ( -1.077988221561493543, -4.724691934501247914, 14.32999329374151465 ) ) ;
#40525=CARTESIAN_POINT ( 'NONE',  ( 2.750000000000001776, -7.499999999999984013, 21.96875000000000355 ) ) ;
#40618=CARTESIAN_POINT ( 'NONE',  ( 2.724691934501250135, -8.700186371490531201, 22.29874329374151642 ) ) ;
#40725=CARTESIAN_POINT ( 'NONE',  ( -2.750000000000007105, -6.360912703474006946, 18.92187500000000355 ) ) ;
#40733=CARTESIAN_POINT ( 'NONE',  ( -2.749999999999991562, -8.639087296526025028, 21.26562500000000000 ) ) ;
#40741=CARTESIAN_POINT ( 'NONE',  ( 1.553300858899087311, -3.749999999999992006, 25.48437500000000000 ) ) ;
#40789=CARTESIAN_POINT ( 'NONE',  ( 3.750000000000000888, -7.499999999999978684, 20.71875000000000000 ) ) ;
#40818=CARTESIAN_POINT ( 'NONE',  ( 2.750000000000001332, -7.438900925035452083, 15.46688170625848713 ) ) ;
#40829=CARTESIAN_POINT ( 'NONE',  ( 2.724691934501235036, -6.299813628509441266, 16.63875670625849068 ) ) ;
#40839=CARTESIAN_POINT ( 'NONE',  ( -3.775308065498748977, -8.992201783934593351, 21.51749329374151998 ) ) ;
#40843=CARTESIAN_POINT ( 'NONE',  ( -3.775308065498748977, -8.992201783934593351, 25.26749329374151642 ) ) ;
#40854=CARTESIAN_POINT ( 'NONE',  ( -2.102533092329708531, -5.360057338231124291, 13.56786352175840626 ) ) ;
#40924=CARTESIAN_POINT ( 'NONE',  ( 1.553300858899129944, -11.24999999999998934, 24.70312500000000000 ) ) ;
#40935=CARTESIAN_POINT ( 'NONE',  ( -1.614399933863656544, -3.775308065498769405, 17.57625670625849068 ) ) ;
#40949=CARTESIAN_POINT ( 'NONE',  ( 1.200186371490529202, -4.775308065498752974, 19.48624329374152353 ) ) ;
#40956=CARTESIAN_POINT ( 'NONE',  ( 1.799775606325937360E-14, -10.25000000000000000, 24.78125000000000000 ) ) ;
#41055=CARTESIAN_POINT ( 'NONE',  ( 1.987747218494642309, -5.598659921968629050, 18.31436829374150932 ) ) ;
#41160=CARTESIAN_POINT ( 'NONE',  ( 1.799775606325937360E-14, -10.25000000000000000, 18.53125000000000000 ) ) ;
#41168=CARTESIAN_POINT ( 'NONE',  ( -1.139087296525992166, -10.25000000000000533, 22.35937500000000711 ) ) ;
#41176=CARTESIAN_POINT ( 'NONE',  ( -3.749999999999997335, -7.500000000000021316, 26.34375000000000000 ) ) ;
#41210=PRODUCT_DEFINITION_SHAPE ( 'NONE', 'NONE',  #47945 ) ;
#41230=CARTESIAN_POINT ( 'NONE',  ( -2.651650429449565305, -4.848349570550461785, 21.50000000000000000 ) ) ;
#41261=CARTESIAN_POINT ( 'NONE',  ( 1.200186371490561621, -10.22469193450123193, 18.20125670625849068 ) ) ;
#41273=CARTESIAN_POINT ( 'NONE',  ( 1.200186371490561621, -10.22469193450123193, 18.20125670625849068 ) ) ;
#41282=CARTESIAN_POINT ( 'NONE',  ( 2.694853999681185108, -4.891553140782077591, 22.06436829374151287 ) ) ;
#41290=CARTESIAN_POINT ( 'NONE',  ( 1.553300858899087311, -3.749999999999992006, 14.23437500000000355 ) ) ;
#41368=CARTESIAN_POINT ( 'NONE',  ( 3.775308065498768517, -8.992201783934554271, 15.54500670625849246 ) ) ;
#41377=CARTESIAN_POINT ( 'NONE',  ( 2.608446859217893099, -4.805146000318787358, 15.31063170625849068 ) ) ;
#41391=CARTESIAN_POINT ( 'NONE',  ( 2.775308065498755195, -6.422011778438505125, 22.14249329374151998 ) ) ;
#41400=CARTESIAN_POINT ( 'NONE',  ( -2.749999999999991562, -8.639087296526026805, 26.26562500000000000 ) ) ;
#41494=CARTESIAN_POINT ( 'NONE',  ( -1.077988221561493543, -4.724691934501247914, 19.32999329374151642 ) ) ;
#41601=CARTESIAN_POINT ( 'NONE',  ( 1.944543648262996083, -5.555456351736983045, 16.81250000000000000 ) ) ;
#41611=CARTESIAN_POINT ( 'NONE',  ( 1.944543648263018731, -9.444543648262994751, 18.37500000000000355 ) ) ;
#41671=CARTESIAN_POINT ( 'NONE',  ( -3.749999999999997335, -7.500000000000021316, 21.34375000000000000 ) ) ;
#41699=CARTESIAN_POINT ( 'NONE',  ( 2.775308065498768517, -8.577988221561467341, 16.79500670625849068 ) ) ;
#41712=CARTESIAN_POINT ( 'NONE',  ( -1.987747218494660295, -5.598659921968651254, 18.74813170625849068 ) ) ;
#41725=CARTESIAN_POINT ( 'NONE',  ( -2.694853999681181556, -10.10844685921792241, 25.18936829374151642 ) ) ;
#41731=CARTESIAN_POINT ( 'NONE',  ( 1.553300858899129944, -11.24999999999998934, 14.70312500000000355 ) ) ;
#41817=CARTESIAN_POINT ( 'NONE',  ( -2.651650429449535551, -10.15165042944956753, 24.93750000000000000 ) ) ;
#41825=CARTESIAN_POINT ( 'NONE',  ( -3.749999999999997335, -7.500000000000021316, 26.34375000000000000 ) ) ;
#41840=CARTESIAN_POINT ( 'NONE',  ( 1.200186371490529202, -4.775308065498752974, 23.23624329374151642 ) ) ;
#41929=CARTESIAN_POINT ( 'NONE',  ( -1.553300858899125059, -3.750000000000009326, 14.07812500000000178 ) ) ;
#41944=CARTESIAN_POINT ( 'NONE',  ( 1.614399933863618797, -3.775308065498751198, 14.48624329374151465 ) ) ;
#42053=CARTESIAN_POINT ( 'NONE',  ( -1.409462824231155764E-14, -4.749999999999999112, 24.15625000000000000 ) ) ;
#42057=( BOUNDED_CURVE ( )  B_SPLINE_CURVE ( 2, ( #45306, #11990, #52946, #17854, #66019, #59270, #25932, #11538, #86775, #60155, #53398, #80899, #25045, #11090, #18742, #52509, #19180, #37668, #86326, #87215, #65129, #3433, #31360, #72778, #25493, #65575, #58368, #66482, #52064, #85863, #4783, #39466, #4328, #39021, #24147, #3875, #51600, #31816, #80448, #58821, #79992, #79556, #79099, #72337, #17405, #46208, #18291, #32257, #73694, #10647, #38112, #83103, #39908, #61485, #62365, #33133, #20506, #6994, #13748, #54726, #239, #47525, #61047, #54280, #81337, #82670, #27704, #12861, #88549, #28145, #82218, #5661, #48412, #55172, #69137, #19617, #40345, #46651, #75020, #26828, #81777, #20064, #75894, #67811, #61925, #47969, #40789, #75452, #20942, #88990, #7445, #74572, #74125, #13307, #41671, #68254, #41230, #68691, #12422, #34464, #88115, #14192, #6114, #60599, #34900, #67368, #26383, #6556, #34018, #27263, #678, #53849, #47082, #33587, #55614, #43441, #28602, #15530, #63702, #30366, #70915, #29931, #36247, #2874, #29056, #14638, #49746, #56512, #56064, #21394, #48860, #70471, #63261, #83555, #23164, #21839, #83997, #69577, #22281, #77220, #16407, #42998, #50631, #2438, #8775, #2009, #29489, #64575, #22714, #56944, #43876, #71343, #57837, #84440, #50177, #57387, #77661, #76333, #42124, #35807, #9220 ),
 .UNSPECIFIED., .F., .F. ) 
 B_SPLINE_CURVE_WITH_KNOTS ( ( 3, 2, 2, 2, 2, 2, 2, 2, 2, 2, 2, 2, 2, 2, 2, 2, 2, 2, 2, 2, 2, 2, 2, 2, 2, 2, 2, 2, 2, 2, 2, 2, 2, 2, 2, 2, 2, 2, 2, 2, 2, 2, 2, 2, 2, 2, 2, 2, 2, 2, 2, 2, 2, 2, 2, 2, 2, 2, 2, 2, 2, 2, 2, 2, 2, 2, 2, 2, 2, 2, 2, 2, 2, 2, 2, 2, 2, 2, 2, 2, 3 ),
 ( 0.000000000000000000, 0.01250000000000000069, 0.02500000000000000139, 0.03749999999999999861, 0.05000000000000000278, 0.06250000000000000000, 0.07499999999999999722, 0.08749999999999999445, 0.1000000000000000056, 0.1125000000000000028, 0.1250000000000000000, 0.1375000000000000111, 0.1499999999999999944, 0.1625000000000000056, 0.1749999999999999889, 0.1875000000000000000, 0.2000000000000000111, 0.2124999999999999944, 0.2250000000000000056, 0.2374999999999999889, 0.2500000000000000000, 0.2625000000000000111, 0.2750000000000000222, 0.2874999999999999778, 0.2999999999999999889, 0.3125000000000000000, 0.3250000000000000111, 0.3375000000000000222, 0.3499999999999999778, 0.3624999999999999889, 0.3750000000000000000, 0.3875000000000000111, 0.4000000000000000222, 0.4124999999999999778, 0.4249999999999999889, 0.4375000000000000000, 0.4500000000000000111, 0.4625000000000000222, 0.4749999999999999778, 0.4874999999999999889, 0.5000000000000000000, 0.5124999999999999556, 0.5250000000000000222, 0.5374999999999999778, 0.5500000000000000444, 0.5625000000000000000, 0.5749999999999999556, 0.5875000000000000222, 0.5999999999999999778, 0.6125000000000000444, 0.6250000000000000000, 0.6374999999999999556, 0.6500000000000000222, 0.6624999999999999778, 0.6750000000000000444, 0.6875000000000000000, 0.6999999999999999556, 0.7125000000000000222, 0.7249999999999999778, 0.7375000000000000444, 0.7500000000000000000, 0.7624999999999999556, 0.7750000000000000222, 0.7874999999999999778, 0.8000000000000000444, 0.8125000000000000000, 0.8249999999999999556, 0.8375000000000000222, 0.8499999999999999778, 0.8625000000000000444, 0.8750000000000000000, 0.8874999999999999556, 0.9000000000000000222, 0.9124999999999999778, 0.9250000000000000444, 0.9375000000000000000, 0.9499999999999999556, 0.9625000000000000222, 0.9749999999999999778, 0.9875000000000000444, 1.000000000000000000 ),
 .UNSPECIFIED. ) 
 CURVE ( )  GEOMETRIC_REPRESENTATION_ITEM ( )  RATIONAL_B_SPLINE_CURVE ( ( 1.000000000000000000, 0.9238795325112867385, 1.000000000000000000, 0.9238795325112867385, 1.000000000000000000, 0.9238795325112867385, 1.000000000000000000, 0.9238795325112867385, 1.000000000000000000, 0.9238795325112867385, 1.000000000000000000, 0.9238795325112867385, 1.000000000000000000, 0.9238795325112867385, 1.000000000000000000, 0.9238795325112867385, 1.000000000000000000, 0.9238795325112867385, 1.000000000000000000, 0.9238795325112867385, 1.000000000000000000, 0.9238795325112867385, 1.000000000000000000, 0.9238795325112867385, 1.000000000000000000, 0.9238795325112867385, 1.000000000000000000, 0.9238795325112867385, 1.000000000000000000, 0.9238795325112867385, 1.000000000000000000, 0.9238795325112867385, 1.000000000000000000, 0.9238795325112867385, 1.000000000000000000, 0.9238795325112867385, 1.000000000000000000, 0.9238795325112867385, 1.000000000000000000, 0.9238795325112867385, 1.000000000000000000, 0.9238795325112867385, 1.000000000000000000, 0.9238795325112867385, 1.000000000000000000, 0.9238795325112867385, 1.000000000000000000, 0.9238795325112867385, 1.000000000000000000, 0.9238795325112867385, 1.000000000000000000, 0.9238795325112867385, 1.000000000000000000, 0.9238795325112867385, 1.000000000000000000, 0.9238795325112867385, 1.000000000000000000, 0.9238795325112867385, 1.000000000000000000, 0.9238795325112867385, 1.000000000000000000, 0.9238795325112867385, 1.000000000000000000, 0.9238795325112867385, 1.000000000000000000, 0.9238795325112867385, 1.000000000000000000, 0.9238795325112867385, 1.000000000000000000, 0.9238795325112867385, 1.000000000000000000, 0.9238795325112867385, 1.000000000000000000, 0.9238795325112867385, 1.000000000000000000, 0.9238795325112867385, 1.000000000000000000, 0.9238795325112867385, 1.000000000000000000, 0.9238795325112867385, 1.000000000000000000, 0.9238795325112867385, 1.000000000000000000, 0.9238795325112867385, 1.000000000000000000, 0.9238795325112867385, 1.000000000000000000, 0.9238795325112867385, 1.000000000000000000, 0.9238795325112867385, 1.000000000000000000, 0.9238795325112867385, 1.000000000000000000, 0.9238795325112867385, 1.000000000000000000, 0.9238795325112867385, 1.000000000000000000, 0.9238795325112867385, 1.000000000000000000, 0.9238795325112867385, 1.000000000000000000, 0.9238795325112867385, 1.000000000000000000, 0.9238795325112867385, 1.000000000000000000, 0.9238795325112867385, 1.000000000000000000, 0.9238795325112867385, 1.000000000000000000, 0.9238795325112867385, 1.000000000000000000, 0.9238795325112867385, 1.000000000000000000, 0.9238795325112867385, 1.000000000000000000, 0.9238795325112867385, 1.000000000000000000, 0.9238795325112867385, 1.000000000000000000, 0.9238795325112867385, 1.000000000000000000, 0.9238795325112867385, 1.000000000000000000, 0.9238795325112867385, 1.000000000000000000, 0.9238795325112867385, 1.000000000000000000, 0.9238795325112867385, 1.000000000000000000, 0.9238795325112867385, 1.000000000000000000, 0.9238795325112867385, 1.000000000000000000, 0.9238795325112867385, 1.000000000000000000, 0.9238795325112867385, 1.000000000000000000, 0.9238795325112867385, 1.000000000000000000, 0.9238795325112867385, 1.000000000000000000, 0.9238795325112867385, 1.000000000000000000, 0.9238795325112867385, 1.000000000000000000, 0.9238795325112867385, 1.000000000000000000, 0.9238795325112867385, 1.000000000000000000, 0.9238795325112867385, 1.000000000000000000, 0.9238795325112867385, 1.000000000000000000, 0.9238795325112867385, 1.000000000000000000, 0.9238795325112867385, 1.000000000000000000, 0.9238795325112867385, 1.000000000000000000, 0.9238795325112867385, 1.000000000000000000 ) ) 
 REPRESENTATION_ITEM ( '' )  );
#42071=CARTESIAN_POINT ( 'NONE',  ( -3.749999999999988454, -9.053300858899127945, 25.01562500000000000 ) ) ;
#42124=CARTESIAN_POINT ( 'NONE',  ( -3.749999999999997335, -7.500000000000021316, 26.34375000000000000 ) ) ;
#42154=CARTESIAN_POINT ( 'NONE',  ( -1.200186371490556958, -4.775308065498765409, 20.07625670625849068 ) ) ;
#42166=CARTESIAN_POINT ( 'NONE',  ( -2.749999999999997780, -7.561099074964547917, 21.09188170625849068 ) ) ;
#42176=CARTESIAN_POINT ( 'NONE',  ( -3.724691934501248802, -5.885600066136383646, 25.42374329374151998 ) ) ;
#42180=CARTESIAN_POINT ( 'NONE',  ( -1.614399933863613468, -11.22469193450124969, 23.86124329374151998 ) ) ;
#42261=CARTESIAN_POINT ( 'NONE',  ( -3.749999999999997335, -7.500000000000021316, 26.34375000000000000 ) ) ;
#42271=CARTESIAN_POINT ( 'NONE',  ( 1.553300858899129944, -11.24999999999998934, 25.95312500000000000 ) ) ;
#42287=CARTESIAN_POINT ( 'NONE',  ( -1.200186371490524317, -10.22469193450124791, 21.36124329374151642 ) ) ;
#42395=CARTESIAN_POINT ( 'NONE',  ( -2.608446859217920633, -4.805146000318815780, 13.00186829374151465 ) ) ;
#42396=ORIENTED_EDGE ( 'NONE', *, *, #28390, .F. ) ;
#42493=CARTESIAN_POINT ( 'NONE',  ( -2.749999999999998224, -7.500000000000015987, 26.34375000000000000 ) ) ;
#42592=CARTESIAN_POINT ( 'NONE',  ( 0.06109907496454976272, -10.25000000000000000, 22.02938170625849068 ) ) ;
#42605=CARTESIAN_POINT ( 'NONE',  ( -1.077988221561460236, -10.27530806549876452, 24.60750670625849779 ) ) ;
#42612=CARTESIAN_POINT ( 'NONE',  ( 3.749999999999992006, -5.946699141100872943, 18.14062500000000711 ) ) ;
#42617=CARTESIAN_POINT ( 'NONE',  ( -3.724691934501248802, -5.885600066136383646, 22.92374329374151998 ) ) ;
#42630=CARTESIAN_POINT ( 'NONE',  ( -2.298097038856290464, -5.201902961143733961, 14.00000000000000000 ) ) ;
#42700=CARTESIAN_POINT ( 'NONE',  ( 3.749999999999999556, -7.438900925035446754, 21.71688170625848713 ) ) ;
#42709=CARTESIAN_POINT ( 'NONE',  ( -3.749999999999996447, -7.561099074964554134, 16.09188170625848713 ) ) ;
#42725=CARTESIAN_POINT ( 'NONE',  ( -2.724691934501246582, -6.299813628509474128, 19.17374329374151642 ) ) ;
#42818=FACE_OUTER_BOUND ( 'NONE', #69495, .T. ) ;
#42830=CARTESIAN_POINT ( 'NONE',  ( -0.06109907496450878162, -11.25000000000000000, 13.78311829374151287 ) ) ;
#42837=CARTESIAN_POINT ( 'NONE',  ( 1.944543648263018731, -9.444543648262994751, 15.87500000000000000 ) ) ;
#42936=CARTESIAN_POINT ( 'NONE',  ( 1.139087296525997273, -4.749999999999992895, 24.23437500000000355 ) ) ;
#42998=CARTESIAN_POINT ( 'NONE',  ( -3.749999999999988454, -9.053300858899127945, 25.01562500000000000 ) ) ;
#43030=CARTESIAN_POINT ( 'NONE',  ( -1.987747218494660295, -5.598659921968651254, 22.49813170625848713 ) ) ;
#43040=CARTESIAN_POINT ( 'NONE',  ( -2.749999999999997780, -7.561099074964547917, 23.59188170625849068 ) ) ;
#43048=CARTESIAN_POINT ( 'NONE',  ( -1.553300858899125059, -3.750000000000009326, 14.07812500000000178 ) ) ;
#43052=CARTESIAN_POINT ( 'NONE',  ( -1.553300858899081538, -11.25000000000000711, 18.60937500000000355 ) ) ;
#43138=CARTESIAN_POINT ( 'NONE',  ( 2.608446859217893099, -4.805146000318787358, 21.56063170625849068 ) ) ;
#43146=CARTESIAN_POINT ( 'NONE',  ( 2.694853999681214862, -10.10844685921789043, 20.62313170625849068 ) ) ;
#43160=CARTESIAN_POINT ( 'NONE',  ( -1.901340078031369618, -5.512252781505359245, 24.25186829374150932 ) ) ;
#43240=CARTESIAN_POINT ( 'NONE',  ( 2.651650429449539104, -4.848349570550432475, 16.81250000000000000 ) ) ;
#43252=CARTESIAN_POINT ( 'NONE',  ( 2.651650429449569302, -10.15165042944953733, 15.87500000000000000 ) ) ;
#43266=CARTESIAN_POINT ( 'NONE',  ( -1.492201783934593573, -3.724691934501250135, 14.32999329374151465 ) ) ;
#43271=CARTESIAN_POINT ( 'NONE',  ( 1.944543648262996083, -5.555456351736983045, 21.81250000000000000 ) ) ;
#43369=CARTESIAN_POINT ( 'NONE',  ( 1.944543648262996083, -5.555456351736983045, 21.81250000000000000 ) ) ;
#43441=CARTESIAN_POINT ( 'NONE',  ( 1.553300858899086867, -3.749999999999992006, 22.98437500000000000 ) ) ;
#43470=CARTESIAN_POINT ( 'NONE',  ( -2.749999999999997780, -7.561099074964547917, 22.34188170625849068 ) ) ;
#43482=CARTESIAN_POINT ( 'NONE',  ( -2.724691934501232371, -8.700186371490559623, 24.76375670625848713 ) ) ;
#43490=CARTESIAN_POINT ( 'NONE',  ( 2.651650429449539104, -4.848349570550432475, 14.31250000000000000 ) ) ;
#43496=CARTESIAN_POINT ( 'NONE',  ( -1.553300858899081538, -11.25000000000000711, 14.85937500000000355 ) ) ;
#43529=CARTESIAN_POINT ( 'NONE',  ( 3.750000000000000888, -7.499999999999978684, 19.46875000000000000 ) ) ;
#43570=CARTESIAN_POINT ( 'NONE',  ( -2.608446859217889546, -10.19485399968121264, 18.43563170625848713 ) ) ;
#43579=CARTESIAN_POINT ( 'NONE',  ( 3.775308065498768517, -8.992201783934554271, 19.29500670625849068 ) ) ;
#43594=CARTESIAN_POINT ( 'NONE',  ( 0.06109907496451268821, -3.749999999999999556, 14.40811829374151110 ) ) ;
#43601=CARTESIAN_POINT ( 'NONE',  ( -2.750000000000006217, -6.360912703474006946, 26.42187500000000000 ) ) ;
#43672=CARTESIAN_POINT ( 'NONE',  ( -2.651650429449565305, -4.848349570550461785, 17.75000000000000355 ) ) ;
#43685=CARTESIAN_POINT ( 'NONE',  ( -1.553300858899125059, -3.750000000000009326, 17.82812500000000000 ) ) ;
#43698=CARTESIAN_POINT ( 'NONE',  ( -1.901340078031369618, -5.512252781505359245, 24.25186829374150932 ) ) ;
#43702=CARTESIAN_POINT ( 'NONE',  ( -1.139087296526025916, -4.750000000000006217, 25.32812500000000711 ) ) ;
#43804=CARTESIAN_POINT ( 'NONE',  ( -1.139087296526025916, -4.750000000000006217, 22.82812500000000355 ) ) ;
#43876=CARTESIAN_POINT ( 'NONE',  ( 3.750000000000000888, -7.499999999999978684, 25.71875000000000000 ) ) ;
#43911=CARTESIAN_POINT ( 'NONE',  ( 0.06109907496454976272, -10.25000000000000000, 20.77938170625848713 ) ) ;
#43914=CARTESIAN_POINT ( 'NONE',  ( 3.205095948332795430, -8.038739123764113259, 14.00000000000000355 ) ) ;
#43921=CARTESIAN_POINT ( 'NONE',  ( 1.987747218494664292, -9.401340078031346081, 24.37313170625848713 ) ) ;
#43929=CARTESIAN_POINT ( 'NONE',  ( 1.553300858899087311, -3.749999999999992006, 17.98437500000000000 ) ) ;
#43934=CARTESIAN_POINT ( 'NONE',  ( 1.553300858899087311, -3.749999999999992006, 16.73437500000000000 ) ) ;
#43970=CARTESIAN_POINT ( 'NONE',  ( 2.320192649118979489E-14, -11.25000000000000000, 21.03125000000000000 ) ) ;
#44008=CARTESIAN_POINT ( 'NONE',  ( -3.749999999999996447, -7.561099074964554134, 19.84188170625848713 ) ) ;
#44017=CARTESIAN_POINT ( 'NONE',  ( 3.749999999999999556, -7.438900925035446754, 22.96688170625849068 ) ) ;
#44030=CARTESIAN_POINT ( 'NONE',  ( 0.06109907496451268821, -3.749999999999999556, 15.65811829374151287 ) ) ;
#44102=CARTESIAN_POINT ( 'NONE',  ( -1.553300858899125059, -3.750000000000009326, 15.32812500000000355 ) ) ;
#44113=CARTESIAN_POINT ( 'NONE',  ( -2.651650429449535551, -10.15165042944956753, 19.93750000000000000 ) ) ;
#44126=CARTESIAN_POINT ( 'NONE',  ( -1.614399933863613468, -11.22469193450124969, 17.61124329374151642 ) ) ;
#44131=CARTESIAN_POINT ( 'NONE',  ( 2.750000000000002665, -7.561099074964516831, 13.47061829374151465 ) ) ;
#44136=CARTESIAN_POINT ( 'NONE',  ( -1.409462824231155764E-14, -4.749999999999999112, 19.15625000000000000 ) ) ;
#44226=CARTESIAN_POINT ( 'NONE',  ( -2.749999999999999112, -7.438900925035484057, 16.59561829374151287 ) ) ;
#44337=CARTESIAN_POINT ( 'NONE',  ( -2.775308065498764964, -6.422011778438537988, 23.67000670625849779 ) ) ;
#44347=CARTESIAN_POINT ( 'NONE',  ( 1.200186371490561621, -10.22469193450123193, 24.45125670625849423 ) ) ;
#44355=CARTESIAN_POINT ( 'NONE',  ( 2.651650429449569302, -10.15165042944953733, 14.62500000000000000 ) ) ;
#44360=CARTESIAN_POINT ( 'NONE',  ( 3.749999999999992006, -5.946699141100872943, 16.89062500000000000 ) ) ;
#44398=CARTESIAN_POINT ( 'NONE',  ( 3.750000000000009770, -9.053300858899081760, 22.04687500000000000 ) ) ;
#44438=CARTESIAN_POINT ( 'NONE',  ( 3.724691934501232815, -5.885600066136343678, 19.13875670625849068 ) ) ;
#44448=CARTESIAN_POINT ( 'NONE',  ( 2.608446859217893099, -4.805146000318787358, 21.56063170625849068 ) ) ;
#44463=CARTESIAN_POINT ( 'NONE',  ( -1.614399933863613468, -11.22469193450124969, 16.36124329374151642 ) ) ;
#44545=CARTESIAN_POINT ( 'NONE',  ( -2.651650429449565305, -4.848349570550461785, 16.50000000000000000 ) ) ;
#44554=CARTESIAN_POINT ( 'NONE',  ( 2.320192649118979489E-14, -11.25000000000000000, 17.28125000000000000 ) ) ;
#44568=CARTESIAN_POINT ( 'NONE',  ( -2.694853999681181556, -10.10844685921792241, 17.68936829374151287 ) ) ;
#44573=CARTESIAN_POINT ( 'NONE',  ( -1.944543648262992530, -9.444543648263016067, 24.93750000000000000 ) ) ;
#44580=CARTESIAN_POINT ( 'NONE',  ( -1.139087296526025250, -4.750000000000006217, 17.82812500000000000 ) ) ;
#44676=CARTESIAN_POINT ( 'NONE',  ( 2.750000000000002665, -7.561099074964516831, 15.97061829374151287 ) ) ;
#44788=CARTESIAN_POINT ( 'NONE',  ( -1.944543648263014957, -5.555456351737005249, 15.25000000000000000 ) ) ;
#44798=CARTESIAN_POINT ( 'NONE',  ( -1.409462824231155764E-14, -4.749999999999999112, 16.65625000000000000 ) ) ;
#44807=CARTESIAN_POINT ( 'NONE',  ( 3.750000000000009770, -9.053300858899081760, 19.54687499999999645 ) ) ;
#44851=CARTESIAN_POINT ( 'NONE',  ( -3.749999999999997335, -7.500000000000021316, 21.34375000000000000 ) ) ;
#44892=CARTESIAN_POINT ( 'NONE',  ( -2.608446859217889546, -10.19485399968121264, 25.93563170625849423 ) ) ;
#44902=CARTESIAN_POINT ( 'NONE',  ( -0.06109907496455085213, -3.750000000000000888, 18.90438170625848713 ) ) ;
#44917=CARTESIAN_POINT ( 'NONE',  ( -1.987747218494638313, -9.401340078031370950, 25.18936829374151642 ) ) ;
#44996=CARTESIAN_POINT ( 'NONE',  ( -1.929879867024197893E-14, -3.750000000000000000, 16.65625000000000000 ) ) ;
#45004=CARTESIAN_POINT ( 'NONE',  ( 2.651650429449539104, -4.848349570550432475, 18.06250000000000355 ) ) ;
#45026=CARTESIAN_POINT ( 'NONE',  ( 1.139087296526029469, -10.24999999999999467, 24.70312500000000000 ) ) ;
#45032=CARTESIAN_POINT ( 'NONE',  ( -2.749999999999991562, -8.639087296526026805, 20.01562500000000355 ) ) ;
#45132=CARTESIAN_POINT ( 'NONE',  ( -1.077988221561493543, -4.724691934501247914, 14.32999329374151465 ) ) ;
#45239=CARTESIAN_POINT ( 'NONE',  ( -1.944543648262992530, -9.444543648263016067, 14.93750000000000000 ) ) ;
#45249=CARTESIAN_POINT ( 'NONE',  ( 1.799775606325937360E-14, -10.25000000000000000, 14.78125000000000178 ) ) ;
#45258=CARTESIAN_POINT ( 'NONE',  ( -2.651650429449535551, -10.15165042944956753, 23.68750000000000000 ) ) ;
#45299=CARTESIAN_POINT ( 'NONE',  ( 2.651650429449569302, -10.15165042944953733, 22.12500000000000000 ) ) ;
#45306=CARTESIAN_POINT ( 'NONE',  ( -2.651650429449565305, -4.848349570550461785, 14.00000000000000178 ) ) ;
#45322=CARTESIAN_POINT ( 'NONE',  ( 2.139942661768877041, -5.397466907670289693, 13.88036352175840626 ) ) ;
#45339=CARTESIAN_POINT ( 'NONE',  ( -1.614399933863656544, -3.775308065498769405, 26.32625670625849068 ) ) ;
#45350=CARTESIAN_POINT ( 'NONE',  ( 2.724691934501235036, -6.299813628509441266, 15.38875670625848890 ) ) ;
#45362=CARTESIAN_POINT ( 'NONE',  ( 0.06109907496451268821, -3.749999999999999556, 19.40811829374151287 ) ) ;
#45379=FACE_OUTER_BOUND ( 'NONE', #57279, .T. ) ;
#45445=CARTESIAN_POINT ( 'NONE',  ( 2.651650429449569302, -10.15165042944953733, 22.12500000000000000 ) ) ;
#45456=CARTESIAN_POINT ( 'NONE',  ( -1.929879867024197893E-14, -3.750000000000000000, 21.65625000000000355 ) ) ;
#45477=CARTESIAN_POINT ( 'NONE',  ( 2.750000000000001776, -7.499999999999984013, 23.21875000000000000 ) ) ;
#45483=CARTESIAN_POINT ( 'NONE',  ( -2.749999999999991562, -8.639087296526026805, 21.26562500000000000 ) ) ;
#45580=CARTESIAN_POINT ( 'NONE',  ( 1.077988221561497539, -10.27530806549875386, 17.45499329374151642 ) ) ;
#45605=SURFACE_SIDE_STYLE ('',( #18591 ) ) ;
#45690=CARTESIAN_POINT ( 'NONE',  ( -2.724691934501232371, -8.700186371490559623, 27.26375670625849423 ) ) ;
#45699=CARTESIAN_POINT ( 'NONE',  ( -1.139087296525992166, -10.25000000000000533, 17.35937500000000000 ) ) ;
#45708=CARTESIAN_POINT ( 'NONE',  ( 3.750000000000000888, -7.499999999999978684, 23.21875000000000000 ) ) ;
#45789=CARTESIAN_POINT ( 'NONE',  ( 2.608446859217893099, -4.805146000318787358, 22.81063170625848713 ) ) ;
#45798=CARTESIAN_POINT ( 'NONE',  ( 3.749999999999999556, -7.438900925035446754, 26.71688170625849068 ) ) ;
#45811=CARTESIAN_POINT ( 'NONE',  ( -0.06109907496450878162, -11.25000000000000000, 20.03311829374151287 ) ) ;
#45841=ORIENTED_EDGE ( 'NONE', *, *, #28390, .T. ) ;
#45893=CARTESIAN_POINT ( 'NONE',  ( 2.651650429449539104, -4.848349570550432475, 23.06250000000000000 ) ) ;
#45901=CARTESIAN_POINT ( 'NONE',  ( -1.553300858899081538, -11.25000000000000711, 23.60937500000000711 ) ) ;
#45919=CARTESIAN_POINT ( 'NONE',  ( 1.987747218494642309, -5.598659921968629050, 18.31436829374150932 ) ) ;
#45925=CARTESIAN_POINT ( 'NONE',  ( -1.944543648262992530, -9.444543648263016067, 17.43750000000000000 ) ) ;
#46028=CARTESIAN_POINT ( 'NONE',  ( 1.987747218494642309, -5.598659921968629050, 14.56436829374151287 ) ) ;
#46143=CARTESIAN_POINT ( 'NONE',  ( -2.749999999999998224, -7.500000000000015987, 16.34375000000000000 ) ) ;
#46153=CARTESIAN_POINT ( 'NONE',  ( -1.944543648263014957, -5.555456351737005249, 15.25000000000000000 ) ) ;
#46163=CARTESIAN_POINT ( 'NONE',  ( -2.651650429449565305, -4.848349570550461785, 21.50000000000000000 ) ) ;
#46202=CARTESIAN_POINT ( 'NONE',  ( -1.929879867024197893E-14, -3.750000000000000000, 25.40625000000000000 ) ) ;
#46208=CARTESIAN_POINT ( 'NONE',  ( -3.749999999999988454, -9.053300858899127945, 17.51562500000000000 ) ) ;
#46241=CARTESIAN_POINT ( 'NONE',  ( -3.775308065498766297, -6.007798216065450170, 27.42000670625849068 ) ) ;
#46251=CARTESIAN_POINT ( 'NONE',  ( -0.06109907496455085213, -3.750000000000000888, 25.15438170625849068 ) ) ;
#46258=CARTESIAN_POINT ( 'NONE',  ( -3.724691934501248802, -5.885600066136383646, 17.92374329374151287 ) ) ;
#46266=CARTESIAN_POINT ( 'NONE',  ( -0.06109907496450878162, -11.25000000000000000, 17.53311829374151287 ) ) ;
#46346=CARTESIAN_POINT ( 'NONE',  ( -3.750000000000008438, -5.946699141100917352, 23.92187500000000355 ) ) ;
#46354=CARTESIAN_POINT ( 'NONE',  ( 3.749999999999992006, -5.946699141100872943, 21.89062500000000355 ) ) ;
#46374=CARTESIAN_POINT ( 'NONE',  ( 2.750000000000002665, -7.561099074964516831, 18.47061829374151287 ) ) ;
#46382=CARTESIAN_POINT ( 'NONE',  ( -1.944543648263014957, -5.555456351737005249, 21.50000000000000000 ) ) ;
#46478=CARTESIAN_POINT ( 'NONE',  ( -1.901340078031369618, -5.512252781505359245, 20.50186829374151287 ) ) ;
#46582=CARTESIAN_POINT ( 'NONE',  ( -2.775308065498764964, -6.422011778438537988, 27.42000670625849068 ) ) ;
#46595=CARTESIAN_POINT ( 'NONE',  ( -2.749999999999998224, -7.500000000000015987, 15.09375000000000000 ) ) ;
#46604=CARTESIAN_POINT ( 'NONE',  ( 2.651650429449539104, -4.848349570550432475, 21.81250000000000000 ) ) ;
#46651=CARTESIAN_POINT ( 'NONE',  ( -3.749999999999988454, -9.053300858899127945, 20.01562500000000355 ) ) ;
#46679=CARTESIAN_POINT ( 'NONE',  ( -1.614399933863656544, -3.775308065498769405, 23.82625670625849068 ) ) ;
#46691=CARTESIAN_POINT ( 'NONE',  ( 3.724691934501232815, -5.885600066136343678, 25.38875670625849423 ) ) ;
#46699=CARTESIAN_POINT ( 'NONE',  ( -1.614399933863613468, -11.22469193450124969, 16.36124329374151642 ) ) ;
#46707=CARTESIAN_POINT ( 'NONE',  ( -1.492201783934593573, -3.724691934501250135, 20.57999329374151998 ) ) ;
#46792=CARTESIAN_POINT ( 'NONE',  ( -3.750000000000008438, -5.946699141100917352, 20.17187500000000000 ) ) ;
#46800=CARTESIAN_POINT ( 'NONE',  ( -2.651650429449565305, -4.848349570550461785, 22.75000000000000000 ) ) ;
#46815=CARTESIAN_POINT ( 'NONE',  ( 1.901340078031373171, -9.487747218494639867, 16.12686829374151287 ) ) ;
#46821=CARTESIAN_POINT ( 'NONE',  ( -2.749999999999991562, -8.639087296526026805, 23.76562500000000000 ) ) ;
#46908=CARTESIAN_POINT ( 'NONE',  ( 2.775308065498755195, -6.422011778438505125, 19.64249329374151642 ) ) ;
#47012=CARTESIAN_POINT ( 'NONE',  ( -1.409462824231155764E-14, -4.749999999999999112, 17.90625000000000000 ) ) ;
#47023=CARTESIAN_POINT ( 'NONE',  ( 2.750000000000001776, -7.499999999999984013, 19.46875000000000000 ) ) ;
#47031=CARTESIAN_POINT ( 'NONE',  ( 3.750000000000009770, -9.053300858899081760, 24.54687500000000000 ) ) ;
#47082=CARTESIAN_POINT ( 'NONE',  ( -2.651650429449565305, -4.848349570550461785, 22.75000000000000000 ) ) ;
#47111=CARTESIAN_POINT ( 'NONE',  ( -1.077988221561460236, -10.27530806549876452, 17.10750670625848713 ) ) ;
#47124=CARTESIAN_POINT ( 'NONE',  ( -2.694853999681210865, -4.891553140782108677, 27.49813170625849068 ) ) ;
#47133=CARTESIAN_POINT ( 'NONE',  ( 0.06109907496451268821, -3.749999999999999556, 19.40811829374151287 ) ) ;
#47141=CARTESIAN_POINT ( 'NONE',  ( -0.06109907496450878162, -11.25000000000000000, 21.28311829374151287 ) ) ;
#47225=CARTESIAN_POINT ( 'NONE',  ( 2.651650429449539104, -4.848349570550432475, 21.81250000000000000 ) ) ;
#47235=CARTESIAN_POINT ( 'NONE',  ( -3.750000000000008438, -5.946699141100917352, 23.92187500000000355 ) ) ;
#47253=CARTESIAN_POINT ( 'NONE',  ( 2.724691934501250135, -8.700186371490531201, 16.04874329374151287 ) ) ;
#47259=CARTESIAN_POINT ( 'NONE',  ( 1.944543648262996083, -5.555456351736983045, 24.31250000000000000 ) ) ;
#47313=ORIENTED_EDGE ( 'NONE', *, *, #66135, .F. ) ;
#47354=CARTESIAN_POINT ( 'NONE',  ( -1.901340078031369618, -5.512252781505359245, 21.75186829374151287 ) ) ;
#47359=( LENGTH_UNIT ( ) NAMED_UNIT ( * ) SI_UNIT ( .MILLI., .METRE. ) );
#47458=CARTESIAN_POINT ( 'NONE',  ( -1.944543648263014957, -5.555456351737005249, 20.25000000000000000 ) ) ;
#47466=CARTESIAN_POINT ( 'NONE',  ( -1.944543648263014957, -5.555456351737005249, 17.75000000000000355 ) ) ;
#47474=CARTESIAN_POINT ( 'NONE',  ( -3.750000000000008438, -5.946699141100917352, 25.17187500000000000 ) ) ;
#47525=CARTESIAN_POINT ( 'NONE',  ( -3.749999999999988454, -9.053300858899127945, 18.76562500000000000 ) ) ;
#47560=CARTESIAN_POINT ( 'NONE',  ( -1.077988221561460236, -10.27530806549876452, 18.35750670625849068 ) ) ;
#47573=CARTESIAN_POINT ( 'NONE',  ( 2.724691934501235036, -6.299813628509441266, 20.38875670625849068 ) ) ;
#47583=CARTESIAN_POINT ( 'NONE',  ( -3.749999999999997780, -7.438900925035489387, 22.84561829374151642 ) ) ;
#47590=CARTESIAN_POINT ( 'NONE',  ( -0.06109907496450878162, -11.25000000000000000, 25.03311829374151287 ) ) ;
#47675=CARTESIAN_POINT ( 'NONE',  ( 3.749999999999999556, -7.438900925035446754, 15.46688170625848713 ) ) ;
#47684=CARTESIAN_POINT ( 'NONE',  ( 3.775308065498768517, -8.992201783934554271, 18.04500670625848713 ) ) ;
#47699=CARTESIAN_POINT ( 'NONE',  ( 2.775308065498755195, -6.422011778438505125, 15.89249329374151820 ) ) ;
#47706=CARTESIAN_POINT ( 'NONE',  ( 2.749999999999995115, -6.360912703473971419, 21.89062500000000355 ) ) ;
#47803=CARTESIAN_POINT ( 'NONE',  ( 1.987747218494642309, -5.598659921968629050, 22.06436829374151287 ) ) ;
#47857=CARTESIAN_POINT ( 'NONE',  ( 1.553300858899129944, -11.24999999999998934, 24.70312500000000000 ) ) ;
#47906=CARTESIAN_POINT ( 'NONE',  ( 1.139087296526029469, -10.24999999999999467, 20.95312500000000000 ) ) ;
#47914=CARTESIAN_POINT ( 'NONE',  ( 2.749999999999995115, -6.360912703473971419, 20.64062500000000000 ) ) ;
#47945=PRODUCT_DEFINITION ( 'UNKNOWN', '', #53350, #70807 ) ;
#47969=CARTESIAN_POINT ( 'NONE',  ( 3.749999999999992006, -5.946699141100872943, 20.64062500000000000 ) ) ;
#47999=CARTESIAN_POINT ( 'NONE',  ( 1.987747218494664292, -9.401340078031346081, 15.62313170625848890 ) ) ;
#48012=CARTESIAN_POINT ( 'NONE',  ( 1.987747218494664292, -9.401340078031346081, 20.62313170625849068 ) ) ;
#48020=CARTESIAN_POINT ( 'NONE',  ( 1.614399933863618797, -3.775308065498751198, 24.48624329374151642 ) ) ;
#48026=CARTESIAN_POINT ( 'NONE',  ( 1.492201783934598236, -11.27530806549875031, 23.70499329374151642 ) ) ;
#48062=CYLINDRICAL_SURFACE ( 'NONE', #49662, 3.000000000000000000 ) ;
#48108=CARTESIAN_POINT ( 'NONE',  ( 0.06109907496455496689, -11.24999999999999822, 15.77938170625848890 ) ) ;
#48119=CARTESIAN_POINT ( 'NONE',  ( -0.06109907496455085213, -3.750000000000000888, 17.65438170625849068 ) ) ;
#48135=CARTESIAN_POINT ( 'NONE',  ( -1.901340078031369618, -5.512252781505359245, 19.25186829374151287 ) ) ;
#48142=CARTESIAN_POINT ( 'NONE',  ( 1.799775606325937360E-14, -10.25000000000000000, 26.03125000000000000 ) ) ;
#48224=CARTESIAN_POINT ( 'NONE',  ( 2.320192649118979489E-14, -11.25000000000000000, 14.78125000000000178 ) ) ;
#48239=CARTESIAN_POINT ( 'NONE',  ( -1.200186371490524317, -10.22469193450124791, 20.11124329374151642 ) ) ;
#48245=FILL_AREA_STYLE ('',( #20779 ) ) ;
#48296=CARTESIAN_POINT ( 'NONE',  ( -2.651650429449565305, -4.848349570550461785, 26.50000000000000355 ) ) ;
#48345=CARTESIAN_POINT ( 'NONE',  ( -1.944543648263014957, -5.555456351737005249, 21.50000000000000000 ) ) ;
#48355=CARTESIAN_POINT ( 'NONE',  ( -1.944543648262992530, -9.444543648263016067, 19.93750000000000000 ) ) ;
#48363=CARTESIAN_POINT ( 'NONE',  ( -2.651650429449535551, -10.15165042944956753, 24.93750000000000000 ) ) ;
#48412=CARTESIAN_POINT ( 'NONE',  ( 2.651650429449569302, -10.15165042944953733, 19.62500000000000000 ) ) ;
#48422=AXIS2_PLACEMENT_3D ( 'NONE', #52582, #81410, #80521 ) ;
#48439=CARTESIAN_POINT ( 'NONE',  ( -1.901340078031346525, -9.487747218494661183, 18.43563170625848713 ) ) ;
#48452=CARTESIAN_POINT ( 'NONE',  ( -1.077988221561460236, -10.27530806549876452, 20.85750670625849068 ) ) ;
#48460=CARTESIAN_POINT ( 'NONE',  ( 2.608446859217924629, -10.19485399968118422, 22.37686829374150932 ) ) ;
#48467=CARTESIAN_POINT ( 'NONE',  ( 1.614399933863618797, -3.775308065498751198, 24.48624329374151642 ) ) ;
#48547=CARTESIAN_POINT ( 'NONE',  ( 3.749999999999999556, -7.438900925035446754, 16.71688170625848713 ) ) ;
#48558=CARTESIAN_POINT ( 'NONE',  ( -3.775308065498766297, -6.007798216065450170, 18.67000670625849068 ) ) ;
#48573=CARTESIAN_POINT ( 'NONE',  ( -2.749999999999999112, -7.438900925035484057, 19.09561829374150932 ) ) ;
#48682=CARTESIAN_POINT ( 'NONE',  ( -1.200186371490524317, -10.22469193450124791, 25.11124329374151642 ) ) ;
#48791=CARTESIAN_POINT ( 'NONE',  ( 1.139087296526029469, -10.24999999999999467, 18.45312500000000355 ) ) ;
#48806=CARTESIAN_POINT ( 'NONE',  ( 1.553300858899129944, -11.24999999999998934, 24.70312500000000000 ) ) ;
#48860=CARTESIAN_POINT ( 'NONE',  ( -1.929879867024197893E-14, -3.750000000000000000, 24.15625000000000000 ) ) ;
#48893=CARTESIAN_POINT ( 'NONE',  ( -2.775308065498764964, -6.422011778438537988, 19.92000670625849068 ) ) ;
#48896=CARTESIAN_POINT ( 'NONE',  ( -2.498132331094908398, -4.694831472195803101, 14.00000000000000178 ) ) ;
#48905=CARTESIAN_POINT ( 'NONE',  ( -2.775308065498764964, -6.422011778438537988, 19.92000670625849068 ) ) ;
#48915=CARTESIAN_POINT ( 'NONE',  ( -1.614399933863613468, -11.22469193450124969, 22.61124329374151287 ) ) ;
#48920=CARTESIAN_POINT ( 'NONE',  ( -3.775308065498748977, -8.992201783934593351, 22.76749329374151287 ) ) ;
#49005=CARTESIAN_POINT ( 'NONE',  ( -0.06109907496455085213, -3.750000000000000888, 17.65438170625849068 ) ) ;
#49013=CARTESIAN_POINT ( 'NONE',  ( -2.608446859217889546, -10.19485399968121264, 15.93563170625849068 ) ) ;
#49027=CARTESIAN_POINT ( 'NONE',  ( 1.077988221561497539, -10.27530806549875386, 21.20499329374151998 ) ) ;
#49132=CARTESIAN_POINT ( 'NONE',  ( -2.775308065498752086, -8.577988221561495763, 24.01749329374151287 ) ) ;
#49140=CARTESIAN_POINT ( 'NONE',  ( -2.749999999999991562, -8.639087296526026805, 15.01562500000000178 ) ) ;
#49244=CARTESIAN_POINT ( 'NONE',  ( 1.799775606325937360E-14, -10.25000000000000000, 26.03125000000000000 ) ) ;
#49345=CARTESIAN_POINT ( 'NONE',  ( 0.06109907496454976272, -10.25000000000000000, 24.52938170625849423 ) ) ;
#49357=CARTESIAN_POINT ( 'NONE',  ( 2.750000000000001332, -7.438900925035452083, 21.71688170625848713 ) ) ;
#49364=CARTESIAN_POINT ( 'NONE',  ( 3.750000000000001776, -7.561099074964511502, 24.72061829374150932 ) ) ;
#49368=CARTESIAN_POINT ( 'NONE',  ( -3.775308065498748977, -8.992201783934593351, 24.01749329374151287 ) ) ;
#49452=CARTESIAN_POINT ( 'NONE',  ( 2.608446859217893099, -4.805146000318787358, 20.31063170625848713 ) ) ;
#49461=CARTESIAN_POINT ( 'NONE',  ( 0.06109907496455496689, -11.24999999999999822, 17.02938170625848713 ) ) ;
#49476=CARTESIAN_POINT ( 'NONE',  ( 2.750000000000002665, -7.561099074964516831, 19.72061829374151287 ) ) ;
#49578=CARTESIAN_POINT ( 'NONE',  ( 1.492201783934598236, -11.27530806549875031, 13.70499329374151287 ) ) ;
#49662=AXIS2_PLACEMENT_3D ( 'NONE', #339, #26481, #27803 ) ;
#49680=CARTESIAN_POINT ( 'NONE',  ( -2.749999999999998224, -7.500000000000015987, 22.59375000000000355 ) ) ;
#49746=CARTESIAN_POINT ( 'NONE',  ( -3.749999999999997335, -7.500000000000021316, 23.84375000000000000 ) ) ;
#49777=CARTESIAN_POINT ( 'NONE',  ( 1.987747218494664292, -9.401340078031346081, 20.62313170625849068 ) ) ;
#49779=CARTESIAN_POINT ( 'NONE',  ( -0.7781152905427543010, -3.838812988065675835, 13.99999999999999289 ) ) ;
#49789=CARTESIAN_POINT ( 'NONE',  ( -1.200186371490556958, -4.775308065498765409, 21.32625670625849423 ) ) ;
#49797=CARTESIAN_POINT ( 'NONE',  ( 2.651650429449539104, -4.848349570550432475, 18.06250000000000355 ) ) ;
#49801=CARTESIAN_POINT ( 'NONE',  ( 3.749999999999992006, -5.946699141100872943, 18.14062500000000711 ) ) ;
#49883=CARTESIAN_POINT ( 'NONE',  ( -3.775308065498766297, -6.007798216065450170, 18.67000670625849068 ) ) ;
#49891=CARTESIAN_POINT ( 'NONE',  ( -2.608446859217889546, -10.19485399968121264, 20.93563170625849068 ) ) ;
#49906=CARTESIAN_POINT ( 'NONE',  ( -0.06109907496451398579, -10.25000000000000178, 21.28311829374151287 ) ) ;
#49987=CARTESIAN_POINT ( 'NONE',  ( -1.929879867024197893E-14, -3.750000000000000000, 15.40625000000000000 ) ) ;
#49997=CARTESIAN_POINT ( 'NONE',  ( -3.749999999999988454, -9.053300858899127945, 18.76562500000000000 ) ) ;
#50014=CARTESIAN_POINT ( 'NONE',  ( -1.987747218494638313, -9.401340078031370950, 25.18936829374151642 ) ) ;
#50019=CARTESIAN_POINT ( 'NONE',  ( -1.139087296525992166, -10.25000000000000533, 19.85937500000000355 ) ) ;
#50115=CARTESIAN_POINT ( 'NONE',  ( 2.749999999999995115, -6.360912703473971419, 25.64062500000000000 ) ) ;
#50177=CARTESIAN_POINT ( 'NONE',  ( 2.320192649118979489E-14, -11.25000000000000000, 26.03125000000000000 ) ) ;
#50208=CARTESIAN_POINT ( 'NONE',  ( 2.775308065498768517, -8.577988221561467341, 24.29500670625849423 ) ) ;
#50211=CARTESIAN_POINT ( 'NONE',  ( 2.705532133667545747, -5.066125464207517304, 14.00000000000000355 ) ) ;
#50220=CARTESIAN_POINT ( 'NONE',  ( -1.987747218494660295, -5.598659921968651254, 22.49813170625848713 ) ) ;
#50227=CARTESIAN_POINT ( 'NONE',  ( -3.750000000000008438, -5.946699141100917352, 16.42187500000000000 ) ) ;
#50231=CARTESIAN_POINT ( 'NONE',  ( -3.750000000000008438, -5.946699141100917352, 16.42187500000000000 ) ) ;
#50234=CARTESIAN_POINT ( 'NONE',  ( -1.944543648263014957, -5.555456351737005249, 26.50000000000000355 ) ) ;
#50270=CARTESIAN_POINT ( 'NONE',  ( 3.750000000000009770, -9.053300858899081760, 19.54687499999999645 ) ) ;
#50316=CARTESIAN_POINT ( 'NONE',  ( -3.775308065498766297, -6.007798216065450170, 19.92000670625849068 ) ) ;
#50326=CARTESIAN_POINT ( 'NONE',  ( 3.724691934501232815, -5.885600066136343678, 22.88875670625849068 ) ) ;
#50340=CARTESIAN_POINT ( 'NONE',  ( 3.750000000000001776, -7.561099074964511502, 13.47061829374151465 ) ) ;
#50422=CARTESIAN_POINT ( 'NONE',  ( 1.553300858899129944, -11.24999999999998934, 15.95312500000000000 ) ) ;
#50435=CARTESIAN_POINT ( 'NONE',  ( 2.651650429449569302, -10.15165042944953733, 17.12500000000000000 ) ) ;
#50450=CARTESIAN_POINT ( 'NONE',  ( -2.724691934501246582, -6.299813628509474128, 25.42374329374151998 ) ) ;
#50454=CARTESIAN_POINT ( 'NONE',  ( -1.139087296525992166, -10.25000000000000533, 24.85937500000001421 ) ) ;
#50558=CARTESIAN_POINT ( 'NONE',  ( -1.944543648263014957, -5.555456351737005249, 26.50000000000000355 ) ) ;
#50631=CARTESIAN_POINT ( 'NONE',  ( -3.749999999999997335, -7.500000000000021316, 25.09374999999999645 ) ) ;
#50659=CARTESIAN_POINT ( 'NONE',  ( -1.987747218494660295, -5.598659921968651254, 24.99813170625849423 ) ) ;
#50661=CARTESIAN_POINT ( 'NONE',  ( 2.248691020740372082, -4.605660251581315201, 14.00000000000000355 ) ) ;
#50668=CARTESIAN_POINT ( 'NONE',  ( 2.775308065498768517, -8.577988221561467341, 23.04500670625849068 ) ) ;
#50675=CARTESIAN_POINT ( 'NONE',  ( -2.608446859217920633, -4.805146000318815780, 25.50186829374151287 ) ) ;
#50679=CARTESIAN_POINT ( 'NONE',  ( -1.553300858899081538, -11.25000000000000711, 17.35937500000000000 ) ) ;
#50716=CARTESIAN_POINT ( 'NONE',  ( 3.750000000000000888, -7.499999999999978684, 23.21875000000000000 ) ) ;
#50755=CARTESIAN_POINT ( 'NONE',  ( 0.06109907496455496689, -11.24999999999999822, 18.27938170625849068 ) ) ;
#50762=CARTESIAN_POINT ( 'NONE',  ( -1.492201783934549164, -11.27530806549876807, 22.10750670625849068 ) ) ;
#50776=CARTESIAN_POINT ( 'NONE',  ( -3.724691934501248802, -5.885600066136383646, 15.42374329374151642 ) ) ;
#50854=CARTESIAN_POINT ( 'NONE',  ( 2.320192649118979489E-14, -11.25000000000000000, 17.28125000000000000 ) ) ;
#50865=CARTESIAN_POINT ( 'NONE',  ( -3.750000000000008438, -5.946699141100917352, 16.42187500000000000 ) ) ;
#50879=CARTESIAN_POINT ( 'NONE',  ( 2.608446859217924629, -10.19485399968118422, 19.87686829374151287 ) ) ;
#50884=CARTESIAN_POINT ( 'NONE',  ( -1.139087296525992166, -10.25000000000000533, 26.10937500000001066 ) ) ;
#50888=CARTESIAN_POINT ( 'NONE',  ( -2.750000000000006217, -6.360912703474006946, 16.42187500000000000 ) ) ;
#50982=CARTESIAN_POINT ( 'NONE',  ( 2.724691934501250135, -8.700186371490531201, 14.79874329374151642 ) ) ;
#51088=CARTESIAN_POINT ( 'NONE',  ( 1.200186371490561621, -10.22469193450123193, 23.20125670625849068 ) ) ;
#51090=CARTESIAN_POINT ( 'NONE',  ( 3.392537894537152265, -7.689361227255397502, 14.00000000000201794 ) ) ;
#51097=CARTESIAN_POINT ( 'NONE',  ( -0.06109907496454585613, -4.750000000000000000, 22.65438170625849068 ) ) ;
#51106=CARTESIAN_POINT ( 'NONE',  ( 2.320192649118979489E-14, -11.25000000000000000, 18.53125000000000000 ) ) ;
#51113=CARTESIAN_POINT ( 'NONE',  ( 3.750000000000000888, -7.499999999999978684, 18.21875000000000000 ) ) ;
#51146=CARTESIAN_POINT ( 'NONE',  ( 1.553300858899129944, -11.24999999999998934, 19.70312500000000355 ) ) ;
#51186=CARTESIAN_POINT ( 'NONE',  ( 2.608446859217893099, -4.805146000318787358, 19.06063170625849068 ) ) ;
#51194=CARTESIAN_POINT ( 'NONE',  ( -2.694853999681210865, -4.891553140782108677, 19.99813170625848713 ) ) ;
#51208=CARTESIAN_POINT ( 'NONE',  ( -3.724691934501248802, -5.885600066136383646, 14.17374329374151287 ) ) ;
#51284=CARTESIAN_POINT ( 'NONE',  ( -2.651650429449565305, -4.848349570550461785, 19.00000000000000000 ) ) ;
#51293=CARTESIAN_POINT ( 'NONE',  ( 1.553300858899129944, -11.24999999999998934, 17.20312500000000000 ) ) ;
#51308=CARTESIAN_POINT ( 'NONE',  ( 1.492201783934598236, -11.27530806549875031, 16.20499329374151642 ) ) ;
#51313=CARTESIAN_POINT ( 'NONE',  ( -1.409462824231155764E-14, -4.749999999999999112, 22.90625000000000355 ) ) ;
#51320=CARTESIAN_POINT ( 'NONE',  ( 2.750000000000001776, -7.499999999999984013, 19.46875000000000000 ) ) ;
#51416=CARTESIAN_POINT ( 'NONE',  ( -1.200186371490524317, -10.22469193450124791, 15.11124329374151287 ) ) ;
#51529=CARTESIAN_POINT ( 'NONE',  ( -1.139087296525992166, -10.25000000000000533, 14.85937500000000355 ) ) ;
#51539=CARTESIAN_POINT ( 'NONE',  ( 1.200186371490561621, -10.22469193450123193, 26.95125670625849068 ) ) ;
#51548=CARTESIAN_POINT ( 'NONE',  ( -2.651650429449535551, -10.15165042944956753, 17.43750000000000000 ) ) ;
#51592=CARTESIAN_POINT ( 'NONE',  ( -2.651650429449535551, -10.15165042944956753, 21.18750000000000000 ) ) ;
#51600=CARTESIAN_POINT ( 'NONE',  ( 2.651650429449539104, -4.848349570550432475, 16.81250000000000000 ) ) ;
#51632=CARTESIAN_POINT ( 'NONE',  ( -1.614399933863656544, -3.775308065498769405, 25.07625670625849423 ) ) ;
#51643=CARTESIAN_POINT ( 'NONE',  ( 2.608446859217893099, -4.805146000318787358, 22.81063170625848713 ) ) ;
#51661=CARTESIAN_POINT ( 'NONE',  ( 2.694853999681185108, -4.891553140782077591, 13.31436829374151287 ) ) ;
#51740=CARTESIAN_POINT ( 'NONE',  ( 3.749999999999992006, -5.946699141100872943, 18.14062500000000711 ) ) ;
#51751=CARTESIAN_POINT ( 'NONE',  ( 2.320192649118979489E-14, -11.25000000000000000, 18.53125000000000000 ) ) ;
#51766=CARTESIAN_POINT ( 'NONE',  ( -3.724691934501248802, -5.885600066136383646, 19.17374329374151642 ) ) ;
#51771=CARTESIAN_POINT ( 'NONE',  ( 1.200186371490529202, -4.775308065498752974, 13.23624329374151465 ) ) ;
#51777=CARTESIAN_POINT ( 'NONE',  ( 1.139087296525997051, -4.749999999999992895, 16.73437500000000000 ) ) ;
#51876=CARTESIAN_POINT ( 'NONE',  ( 1.987747218494642309, -5.598659921968629050, 17.06436829374151287 ) ) ;
#51991=CARTESIAN_POINT ( 'NONE',  ( 2.749999999999995115, -6.360912703473971419, 14.39062500000000178 ) ) ;
#52001=CARTESIAN_POINT ( 'NONE',  ( 1.901340078031349856, -5.512252781505337929, 26.56063170625849068 ) ) ;
#52011=CARTESIAN_POINT ( 'NONE',  ( -1.553300858899125059, -3.750000000000009326, 21.57812500000000355 ) ) ;
#52056=CARTESIAN_POINT ( 'NONE',  ( -1.553300858899081538, -11.25000000000000711, 21.10937500000000711 ) ) ;
#52064=CARTESIAN_POINT ( 'NONE',  ( -2.651650429449535551, -10.15165042944956753, 16.18750000000000000 ) ) ;
#52097=CARTESIAN_POINT ( 'NONE',  ( -3.749999999999996447, -7.561099074964554134, 26.09188170625848358 ) ) ;
#52107=CARTESIAN_POINT ( 'NONE',  ( 0.06109907496455496689, -11.24999999999999822, 24.52938170625849423 ) ) ;
#52121=CARTESIAN_POINT ( 'NONE',  ( -3.775308065498748977, -8.992201783934593351, 20.26749329374151998 ) ) ;
#52201=CARTESIAN_POINT ( 'NONE',  ( -3.749999999999988454, -9.053300858899127945, 21.26562500000000000 ) ) ;
#52211=CARTESIAN_POINT ( 'NONE',  ( 1.553300858899087311, -3.749999999999992006, 21.73437500000000000 ) ) ;
#52229=CARTESIAN_POINT ( 'NONE',  ( -1.987747218494638313, -9.401340078031370950, 13.93936829374151465 ) ) ;
#52236=CARTESIAN_POINT ( 'NONE',  ( 1.799775606325937360E-14, -10.25000000000000000, 21.03125000000000000 ) ) ;
#52266=CARTESIAN_POINT ( 'NONE',  ( -2.298097038856290464, -5.201902961143733961, 26.50000000000000355 ) ) ;
#52331=CARTESIAN_POINT ( 'NONE',  ( -2.724691934501246582, -6.299813628509474128, 15.42374329374151642 ) ) ;
#52440=CARTESIAN_POINT ( 'NONE',  ( 1.901340078031349856, -5.512252781505337929, 25.31063170625848713 ) ) ;
#52449=CARTESIAN_POINT ( 'NONE',  ( 1.799775606325937360E-14, -10.25000000000000000, 17.28125000000000000 ) ) ;
#52458=CARTESIAN_POINT ( 'NONE',  ( -1.553300858899125059, -3.750000000000009326, 19.07812500000000000 ) ) ;
#52501=CARTESIAN_POINT ( 'NONE',  ( -2.651650429449535551, -10.15165042944956753, 24.93750000000000000 ) ) ;
#52509=CARTESIAN_POINT ( 'NONE',  ( -3.750000000000007550, -5.946699141100917352, 15.17187500000000000 ) ) ;
#52541=CARTESIAN_POINT ( 'NONE',  ( 3.724691934501232815, -5.885600066136343678, 26.63875670625848713 ) ) ;
#52551=CARTESIAN_POINT ( 'NONE',  ( 1.987747218494664292, -9.401340078031346081, 15.62313170625848890 ) ) ;
#52564=CARTESIAN_POINT ( 'NONE',  ( 3.724691934501251023, -9.114399933863618131, 19.79874329374151287 ) ) ;
#52582=CARTESIAN_POINT ( 'NONE',  ( 1.653273178848927064E-15, -7.500000000000000000, 14.00000000000000178 ) ) ;
#52650=CARTESIAN_POINT ( 'NONE',  ( 2.320192649118979489E-14, -11.25000000000000000, 22.28125000000000355 ) ) ;
#52658=CARTESIAN_POINT ( 'NONE',  ( 2.320192649118979489E-14, -11.25000000000000000, 21.03125000000000000 ) ) ;
#52676=CARTESIAN_POINT ( 'NONE',  ( 0.06109907496451789238, -4.749999999999998224, 18.15811829374151642 ) ) ;
#52682=CARTESIAN_POINT ( 'NONE',  ( 2.750000000000008438, -8.639087296525996607, 17.04687500000000000 ) ) ;
#52778=CARTESIAN_POINT ( 'NONE',  ( -1.901340078031369618, -5.512252781505359245, 18.00186829374151287 ) ) ;
#52883=CARTESIAN_POINT ( 'NONE',  ( -2.749999999999991562, -8.639087296526025028, 16.26562500000000000 ) ) ;
#52891=CARTESIAN_POINT ( 'NONE',  ( 2.749999999999995115, -6.360912703473971419, 14.39062500000000178 ) ) ;
#52900=CARTESIAN_POINT ( 'NONE',  ( -2.651650429449535551, -10.15165042944956753, 19.93750000000000000 ) ) ;
#52946=CARTESIAN_POINT ( 'NONE',  ( -1.929879867024197893E-14, -3.750000000000000000, 14.15625000000000000 ) ) ;
#52981=CARTESIAN_POINT ( 'NONE',  ( -3.724691934501229262, -9.114399933863657211, 27.26375670625849423 ) ) ;
#52990=CARTESIAN_POINT ( 'NONE',  ( -3.775308065498766297, -6.007798216065450170, 27.42000670625849068 ) ) ;
#53004=CARTESIAN_POINT ( 'NONE',  ( -3.724691934501248802, -5.885600066136383646, 16.67374329374151998 ) ) ;
#53078=CARTESIAN_POINT ( 'NONE',  ( -1.944543648263015179, -5.555456351737005249, 14.00000000000000000 ) ) ;
#53088=CARTESIAN_POINT ( 'NONE',  ( 1.553300858899087311, -3.749999999999992006, 22.98437500000000000 ) ) ;
#53098=CARTESIAN_POINT ( 'NONE',  ( -3.749999999999997335, -7.500000000000021316, 22.59375000000000355 ) ) ;
#53116=CARTESIAN_POINT ( 'NONE',  ( -0.06109907496451398579, -10.25000000000000178, 15.03311829374151287 ) ) ;
#53123=CARTESIAN_POINT ( 'NONE',  ( 2.750000000000008438, -8.639087296525996607, 24.54687500000000000 ) ) ;
#53213=COLOUR_RGB ( '', 0.66274510, 0.83137255, 0.94901961) ;
#53222=CARTESIAN_POINT ( 'NONE',  ( 2.724691934501250135, -8.700186371490531201, 18.54874329374151642 ) ) ;
#53308=CARTESIAN_POINT ( 'NONE',  ( -2.108822856672541768, -5.366237147583038158, 13.71190574791610928 ) ) ;
#53329=CARTESIAN_POINT ( 'NONE',  ( 1.901340078031349856, -5.512252781505337929, 26.56063170625849068 ) ) ;
#53341=CARTESIAN_POINT ( 'NONE',  ( 2.749999999999995115, -6.360912703473971419, 15.64062500000000178 ) ) ;
#53350=PRODUCT_DEFINITION_FORMATION_WITH_SPECIFIED_SOURCE ( 'ANY', '', #54864, .NOT_KNOWN. ) ;
#53351=CARTESIAN_POINT ( 'NONE',  ( -2.651650429449565305, -4.848349570550461785, 22.75000000000000000 ) ) ;
#53398=CARTESIAN_POINT ( 'NONE',  ( 2.320192649118979489E-14, -11.25000000000000000, 14.78125000000000178 ) ) ;
#53426=CARTESIAN_POINT ( 'NONE',  ( 3.724691934501232815, -5.885600066136343678, 24.13875670625849068 ) ) ;
#53437=ORIENTED_EDGE ( 'NONE', *, *, #28885, .T. ) ;
#53440=CARTESIAN_POINT ( 'NONE',  ( -2.694853999681210865, -4.891553140782108677, 24.99813170625849423 ) ) ;
#53447=CARTESIAN_POINT ( 'NONE',  ( 3.724691934501251023, -9.114399933863618131, 19.79874329374151287 ) ) ;
#53454=CARTESIAN_POINT ( 'NONE',  ( -2.694853999681181556, -10.10844685921792241, 20.18936829374151287 ) ) ;
#53538=CARTESIAN_POINT ( 'NONE',  ( -1.929879867024197893E-14, -3.750000000000000000, 24.15625000000000000 ) ) ;
#53550=CARTESIAN_POINT ( 'NONE',  ( -1.553300858899125059, -3.750000000000009326, 20.32812500000000000 ) ) ;
#53567=CARTESIAN_POINT ( 'NONE',  ( 1.077988221561497539, -10.27530806549875386, 18.70499329374151287 ) ) ;
#53574=CARTESIAN_POINT ( 'NONE',  ( -2.749999999999998224, -7.500000000000015987, 25.09374999999999645 ) ) ;
#53674=CARTESIAN_POINT ( 'NONE',  ( 1.987747218494642309, -5.598659921968629050, 19.56436829374151287 ) ) ;
#53740=DIRECTION ( 'NONE',  ( 0.000000000000000000, 0.000000000000000000, 1.000000000000000000 ) ) ;
#53779=CARTESIAN_POINT ( 'NONE',  ( -1.139087296526025916, -4.750000000000006217, 20.32812500000000000 ) ) ;
#53788=CARTESIAN_POINT ( 'NONE',  ( 1.944543648262996083, -5.555456351736983045, 19.31250000000000000 ) ) ;
#53849=CARTESIAN_POINT ( 'NONE',  ( -3.750000000000007550, -5.946699141100917352, 22.67187499999999645 ) ) ;
#53880=CARTESIAN_POINT ( 'NONE',  ( 0.06109907496454976272, -10.25000000000000000, 17.02938170625848713 ) ) ;
#53893=CARTESIAN_POINT ( 'NONE',  ( -3.724691934501229262, -9.114399933863657211, 27.26375670625849423 ) ) ;
#53900=CARTESIAN_POINT ( 'NONE',  ( -0.06109907496450878162, -11.25000000000000000, 18.78311829374151287 ) ) ;
#53906=CARTESIAN_POINT ( 'NONE',  ( 2.608446859217924629, -10.19485399968118422, 21.12686829374151287 ) ) ;
#53988=CARTESIAN_POINT ( 'NONE',  ( 3.750000000000000888, -7.499999999999978684, 19.46875000000000000 ) ) ;
#53996=CARTESIAN_POINT ( 'NONE',  ( -2.651650429449565305, -4.848349570550461785, 25.25000000000000000 ) ) ;
#54009=CARTESIAN_POINT ( 'NONE',  ( -1.077988221561493543, -4.724691934501247914, 16.82999329374151287 ) ) ;
#54014=CARTESIAN_POINT ( 'NONE',  ( -1.139087296526025250, -4.750000000000006217, 21.57812500000000355 ) ) ;
#54106=CARTESIAN_POINT ( 'NONE',  ( 2.724691934501250135, -8.700186371490531201, 19.79874329374151287 ) ) ;
#54213=CARTESIAN_POINT ( 'NONE',  ( 2.749999999999995115, -6.360912703473971419, 16.89062500000000000 ) ) ;
#54223=CARTESIAN_POINT ( 'NONE',  ( 1.139087296525997273, -4.749999999999992895, 21.73437500000000000 ) ) ;
#54230=CARTESIAN_POINT ( 'NONE',  ( 1.553300858899087311, -3.749999999999992006, 24.23437500000000355 ) ) ;
#54280=CARTESIAN_POINT ( 'NONE',  ( -3.750000000000007550, -5.946699141100917352, 18.92187500000000000 ) ) ;
#54314=CARTESIAN_POINT ( 'NONE',  ( 1.987747218494664292, -9.401340078031346081, 19.37313170625848713 ) ) ;
#54327=CARTESIAN_POINT ( 'NONE',  ( 1.077988221561464899, -4.724691934501233703, 20.23250670625849423 ) ) ;
#54334=CARTESIAN_POINT ( 'NONE',  ( 3.724691934501251023, -9.114399933863618131, 22.29874329374151642 ) ) ;
#54340=CARTESIAN_POINT ( 'NONE',  ( 3.750000000000001776, -7.561099074964511502, 24.72061829374150932 ) ) ;
#54426=CARTESIAN_POINT ( 'NONE',  ( -1.492201783934549164, -11.27530806549876807, 17.10750670625848713 ) ) ;
#54435=CARTESIAN_POINT ( 'NONE',  ( 1.553300858899087311, -3.749999999999992006, 25.48437500000000000 ) ) ;
#54451=CARTESIAN_POINT ( 'NONE',  ( -1.901340078031369618, -5.512252781505359245, 15.50186829374151287 ) ) ;
#54457=CARTESIAN_POINT ( 'NONE',  ( 1.139087296525997051, -4.749999999999992895, 25.48437500000000000 ) ) ;
#54550=CARTESIAN_POINT ( 'NONE',  ( -2.775308065498752086, -8.577988221561495763, 22.76749329374151287 ) ) ;
#54558=SURFACE_SIDE_STYLE ('',( #6395 ) ) ;
#54604=CARTESIAN_POINT ( 'NONE',  ( 2.320192649118979489E-14, -11.25000000000000000, 26.03125000000000000 ) ) ;
#54654=CARTESIAN_POINT ( 'NONE',  ( 2.750000000000001776, -7.499999999999984013, 20.71875000000000000 ) ) ;
#54663=CARTESIAN_POINT ( 'NONE',  ( -2.749999999999998224, -7.500000000000015987, 21.34375000000000000 ) ) ;
#54671=CARTESIAN_POINT ( 'NONE',  ( -3.749999999999997335, -7.500000000000021316, 25.09374999999999645 ) ) ;
#54726=CARTESIAN_POINT ( 'NONE',  ( -1.553300858899081760, -11.25000000000000888, 18.60937500000000355 ) ) ;
#54761=CARTESIAN_POINT ( 'NONE',  ( 2.775308065498768517, -8.577988221561467341, 18.04500670625848713 ) ) ;
#54772=CARTESIAN_POINT ( 'NONE',  ( 2.750000000000001332, -7.438900925035452083, 17.96688170625848713 ) ) ;
#54781=CARTESIAN_POINT ( 'NONE',  ( -3.724691934501248802, -5.885600066136383646, 22.92374329374151998 ) ) ;
#54787=CARTESIAN_POINT ( 'NONE',  ( -3.724691934501248802, -5.885600066136383646, 21.67374329374151287 ) ) ;
#54864=PRODUCT ( 'spring', 'spring', '', ( #40156 ) ) ;
#54878=CARTESIAN_POINT ( 'NONE',  ( 3.750000000000009770, -9.053300858899081760, 25.79687500000000355 ) ) ;
#54888=CARTESIAN_POINT ( 'NONE',  ( -2.694853999681210865, -4.891553140782108677, 16.24813170625848713 ) ) ;
#54903=CARTESIAN_POINT ( 'NONE',  ( -2.724691934501246582, -6.299813628509474128, 22.92374329374151998 ) ) ;
#54909=CARTESIAN_POINT ( 'NONE',  ( 2.750000000000008438, -8.639087296525996607, 25.79687500000000355 ) ) ;
#55006=CARTESIAN_POINT ( 'NONE',  ( 2.750000000000002665, -7.561099074964516831, 18.47061829374151287 ) ) ;
#55060=CARTESIAN_POINT ( 'NONE',  ( 3.749999999999992006, -5.946699141100872943, 24.39062500000000000 ) ) ;
#55109=CARTESIAN_POINT ( 'NONE',  ( -2.749999999999991562, -8.639087296526025028, 21.26562500000000000 ) ) ;
#55118=CARTESIAN_POINT ( 'NONE',  ( -2.749999999999991562, -8.639087296526025028, 20.01562500000000355 ) ) ;
#55172=CARTESIAN_POINT ( 'NONE',  ( 1.553300858899129722, -11.24999999999999112, 19.70312500000000355 ) ) ;
#55206=CARTESIAN_POINT ( 'NONE',  ( 0.06109907496454976272, -10.25000000000000000, 15.77938170625848890 ) ) ;
#55219=CARTESIAN_POINT ( 'NONE',  ( -1.987747218494660295, -5.598659921968651254, 19.99813170625848713 ) ) ;
#55227=CARTESIAN_POINT ( 'NONE',  ( -3.775308065498748977, -8.992201783934593351, 22.76749329374151287 ) ) ;
#55232=CARTESIAN_POINT ( 'NONE',  ( -2.608446859217920633, -4.805146000318815780, 23.00186829374151287 ) ) ;
#55297=VERTEX_POINT ( 'NONE', #40854 ) ;
#55312=CARTESIAN_POINT ( 'NONE',  ( -3.724691934501229262, -9.114399933863657211, 16.01375670625849068 ) ) ;
#55323=CARTESIAN_POINT ( 'NONE',  ( -0.06109907496455085213, -3.750000000000000888, 16.40438170625849068 ) ) ;
#55338=CARTESIAN_POINT ( 'NONE',  ( -2.775308065498752086, -8.577988221561495763, 22.76749329374151287 ) ) ;
#55430=CARTESIAN_POINT ( 'NONE',  ( -3.749999999999997335, -7.500000000000021316, 15.09375000000000000 ) ) ;
#55446=CARTESIAN_POINT ( 'NONE',  ( -0.06109907496451398579, -10.25000000000000178, 23.78311829374151998 ) ) ;
#55549=CARTESIAN_POINT ( 'NONE',  ( -1.139087296525992166, -10.25000000000000533, 18.60937500000000355 ) ) ;
#55614=CARTESIAN_POINT ( 'NONE',  ( -1.929879867024197893E-14, -3.750000000000000000, 22.90625000000000355 ) ) ;
#55643=CARTESIAN_POINT ( 'NONE',  ( 2.724691934501235036, -6.299813628509441266, 16.63875670625849068 ) ) ;
#55655=CARTESIAN_POINT ( 'NONE',  ( -2.775308065498764964, -6.422011778438537988, 18.67000670625849068 ) ) ;
#55663=CARTESIAN_POINT ( 'NONE',  ( -3.724691934501248802, -5.885600066136383646, 21.67374329374151287 ) ) ;
#55669=CARTESIAN_POINT ( 'NONE',  ( 0.06109907496451268821, -3.749999999999999556, 21.90811829374151642 ) ) ;
#55754=CARTESIAN_POINT ( 'NONE',  ( -2.694853999681210865, -4.891553140782108677, 17.49813170625848713 ) ) ;
#55763=CARTESIAN_POINT ( 'NONE',  ( 1.492201783934554493, -3.724691934501233703, 16.48250670625849423 ) ) ;
#55777=CARTESIAN_POINT ( 'NONE',  ( 2.775308065498755195, -6.422011778438505125, 23.39249329374151642 ) ) ;
#55886=CARTESIAN_POINT ( 'NONE',  ( -3.724691934501248802, -5.885600066136383646, 15.42374329374151642 ) ) ;
#55896=EDGE_CURVE ( 'NONE', #25338, #76825, #34881, .T. ) ;
#55994=CARTESIAN_POINT ( 'NONE',  ( 1.944543648263018731, -9.444543648262994751, 25.87500000000000355 ) ) ;
#56064=CARTESIAN_POINT ( 'NONE',  ( -2.651650429449565305, -4.848349570550461785, 24.00000000000000000 ) ) ;
#56097=CARTESIAN_POINT ( 'NONE',  ( 1.077988221561464899, -4.724691934501233703, 22.73250670625849068 ) ) ;
#56109=CARTESIAN_POINT ( 'NONE',  ( -1.077988221561460236, -10.27530806549876452, 17.10750670625848713 ) ) ;
#56119=CARTESIAN_POINT ( 'NONE',  ( -2.608446859217920633, -4.805146000318815780, 21.75186829374151287 ) ) ;
#56125=CARTESIAN_POINT ( 'NONE',  ( -2.694853999681181556, -10.10844685921792241, 23.93936829374151642 ) ) ;
#56207=CARTESIAN_POINT ( 'NONE',  ( 3.750000000000000888, -7.499999999999978684, 24.46875000000000000 ) ) ;
#56215=CARTESIAN_POINT ( 'NONE',  ( -3.724691934501229262, -9.114399933863657211, 16.01375670625849068 ) ) ;
#56231=CARTESIAN_POINT ( 'NONE',  ( -1.077988221561493543, -4.724691934501247914, 19.32999329374151642 ) ) ;
#56338=CARTESIAN_POINT ( 'NONE',  ( 2.694853999681185108, -4.891553140782077591, 13.31436829374151287 ) ) ;
#56443=CARTESIAN_POINT ( 'NONE',  ( -2.750000000000007105, -6.360912703474006946, 26.42187500000000000 ) ) ;
#56512=CARTESIAN_POINT ( 'NONE',  ( -3.750000000000007550, -5.946699141100917352, 23.92187500000000355 ) ) ;
#56542=CARTESIAN_POINT ( 'NONE',  ( -2.775308065498764964, -6.422011778438537988, 24.92000670625849068 ) ) ;
#56555=CARTESIAN_POINT ( 'NONE',  ( 1.077988221561464899, -4.724691934501233703, 23.98250670625849068 ) ) ;
#56563=CARTESIAN_POINT ( 'NONE',  ( 2.651650429449539104, -4.848349570550432475, 16.81250000000000000 ) ) ;
#56568=CARTESIAN_POINT ( 'NONE',  ( 3.750000000000009770, -9.053300858899081760, 15.79687500000000178 ) ) ;
#56647=CARTESIAN_POINT ( 'NONE',  ( -3.724691934501229262, -9.114399933863657211, 22.26375670625849068 ) ) ;
#56656=CARTESIAN_POINT ( 'NONE',  ( -3.724691934501229262, -9.114399933863657211, 23.51375670625848713 ) ) ;
#56670=CARTESIAN_POINT ( 'NONE',  ( 0.06109907496451789238, -4.749999999999998224, 23.15811829374151642 ) ) ;
#56749=CARTESIAN_POINT ( 'NONE',  ( 3.750000000000000888, -7.499999999999978684, 15.71875000000000000 ) ) ;
#56771=CARTESIAN_POINT ( 'NONE',  ( 1.200186371490529202, -4.775308065498752974, 24.48624329374151642 ) ) ;
#56775=CARTESIAN_POINT ( 'NONE',  ( -1.409462824231155764E-14, -4.749999999999999112, 21.65625000000000355 ) ) ;
#56779=CARTESIAN_POINT ( 'NONE',  ( 1.139087296526029469, -10.24999999999999289, 14.70312500000000355 ) ) ;
#56875=CARTESIAN_POINT ( 'NONE',  ( 1.139087296525997273, -4.749999999999992895, 22.98437500000000000 ) ) ;
#56944=CARTESIAN_POINT ( 'NONE',  ( 3.749999999999992006, -5.946699141100872943, 25.64062500000000000 ) ) ;
#56976=CARTESIAN_POINT ( 'NONE',  ( -2.724691934501232371, -8.700186371490559623, 24.76375670625848713 ) ) ;
#56979=CARTESIAN_POINT ( 'NONE',  ( 3.443994336716911242, -7.367359615244446935, 14.00000000000001421 ) ) ;
#56989=CARTESIAN_POINT ( 'NONE',  ( 1.901340078031349856, -5.512252781505337929, 24.06063170625849423 ) ) ;
#56997=CARTESIAN_POINT ( 'NONE',  ( -1.553300858899081538, -11.25000000000000711, 14.85937500000000355 ) ) ;
#57001=CARTESIAN_POINT ( 'NONE',  ( 3.750000000000009770, -9.053300858899081760, 17.04687500000000000 ) ) ;
#57041=CARTESIAN_POINT ( 'NONE',  ( -1.553300858899125059, -3.750000000000009326, 22.82812500000000355 ) ) ;
#57084=CARTESIAN_POINT ( 'NONE',  ( -3.749999999999996447, -7.561099074964554134, 18.59188170625849068 ) ) ;
#57093=CARTESIAN_POINT ( 'NONE',  ( -3.775308065498766297, -6.007798216065450170, 23.67000670625849779 ) ) ;
#57111=CARTESIAN_POINT ( 'NONE',  ( 2.775308065498755195, -6.422011778438505125, 24.64249329374151642 ) ) ;
#57193=CARTESIAN_POINT ( 'NONE',  ( -2.651650429449535551, -10.15165042944956753, 17.43750000000000000 ) ) ;
#57205=CARTESIAN_POINT ( 'NONE',  ( 3.749999999999992006, -5.946699141100872943, 19.39062500000000711 ) ) ;
#57221=CARTESIAN_POINT ( 'NONE',  ( 2.775308065498755195, -6.422011778438505125, 23.39249329374151642 ) ) ;
#57225=CARTESIAN_POINT ( 'NONE',  ( 1.799775606325937360E-14, -10.25000000000000000, 23.53125000000000000 ) ) ;
#57229=CARTESIAN_POINT ( 'NONE',  ( -1.944543648262992530, -9.444543648263016067, 16.18750000000000000 ) ) ;
#57234=UNCERTAINTY_MEASURE_WITH_UNIT (LENGTH_MEASURE( 1.000000000000000082E-05 ), #25788, 'distance_accuracy_value', 'NONE');
#57279=EDGE_LOOP ( 'NONE', ( #86230, #67133, #78367 ) ) ;
#57323=CARTESIAN_POINT ( 'NONE',  ( 1.944543648262996083, -5.555456351736983045, 25.56250000000000355 ) ) ;
#57387=CARTESIAN_POINT ( 'NONE',  ( -1.553300858899081760, -11.25000000000000888, 26.10937500000000355 ) ) ;
#57419=CARTESIAN_POINT ( 'NONE',  ( 2.750000000000001332, -7.438900925035452083, 20.46688170625848713 ) ) ;
#57430=CARTESIAN_POINT ( 'NONE',  ( 1.987747218494664292, -9.401340078031346081, 21.87313170625849068 ) ) ;
#57437=CARTESIAN_POINT ( 'NONE',  ( -2.651650429449565305, -4.848349570550461785, 17.75000000000000355 ) ) ;
#57443=CARTESIAN_POINT ( 'NONE',  ( -3.749999999999988454, -9.053300858899127945, 18.76562500000000000 ) ) ;
#57484=CARTESIAN_POINT ( 'NONE',  ( -1.929879867024197893E-14, -3.750000000000000000, 22.90625000000000355 ) ) ;
#57528=CARTESIAN_POINT ( 'NONE',  ( -3.724691934501229262, -9.114399933863657211, 19.76375670625849423 ) ) ;
#57535=CARTESIAN_POINT ( 'NONE',  ( -0.06109907496455085213, -3.750000000000000888, 21.40438170625849068 ) ) ;
#57550=CARTESIAN_POINT ( 'NONE',  ( -3.749999999999997780, -7.438900925035489387, 15.34561829374151465 ) ) ;
#57633=CARTESIAN_POINT ( 'NONE',  ( -2.651650429449535551, -10.15165042944956753, 16.18750000000000000 ) ) ;
#57644=CARTESIAN_POINT ( 'NONE',  ( 3.750000000000009770, -9.053300858899081760, 18.29687500000000000 ) ) ;
#57660=CARTESIAN_POINT ( 'NONE',  ( 1.614399933863618797, -3.775308065498751198, 15.73624329374151998 ) ) ;
#57664=CARTESIAN_POINT ( 'NONE',  ( -1.409462824231155764E-14, -4.749999999999999112, 25.40625000000000000 ) ) ;
#57765=CARTESIAN_POINT ( 'NONE',  ( 2.750000000000008438, -8.639087296525996607, 23.29687500000000000 ) ) ;
#57786=EDGE_LOOP ( 'NONE', ( #939, #70407 ) ) ;
#57837=CARTESIAN_POINT ( 'NONE',  ( 2.651650429449569302, -10.15165042944953733, 25.87500000000000355 ) ) ;
#57868=CARTESIAN_POINT ( 'NONE',  ( 2.724691934501235036, -6.299813628509441266, 22.88875670625849068 ) ) ;
#57870=CARTESIAN_POINT ( 'NONE',  ( 3.299694722263635693, -7.944920208824736818, 14.00000000000000178 ) ) ;
#57877=CARTESIAN_POINT ( 'NONE',  ( -2.724691934501232371, -8.700186371490559623, 26.01375670625848713 ) ) ;
#57885=CARTESIAN_POINT ( 'NONE',  ( -3.749999999999997335, -7.500000000000021316, 16.34375000000000000 ) ) ;
#57889=CARTESIAN_POINT ( 'NONE',  ( 2.651650429449569302, -10.15165042944953733, 17.12500000000000000 ) ) ;
#57929=CARTESIAN_POINT ( 'NONE',  ( -3.749999999999988454, -9.053300858899127945, 23.76562499999999645 ) ) ;
#57970=CARTESIAN_POINT ( 'NONE',  ( -1.492201783934549164, -11.27530806549876807, 22.10750670625849068 ) ) ;
#57978=CARTESIAN_POINT ( 'NONE',  ( -1.614399933863656544, -3.775308065498769405, 18.82625670625848713 ) ) ;
#57994=CARTESIAN_POINT ( 'NONE',  ( 3.775308065498752086, -6.007798216065404873, 13.39249329374151642 ) ) ;
#58071=CARTESIAN_POINT ( 'NONE',  ( 2.320192649118979489E-14, -11.25000000000000000, 14.78125000000000178 ) ) ;
#58074=VERTEX_POINT ( 'NONE', #20153 ) ;
#58082=CARTESIAN_POINT ( 'NONE',  ( 1.553300858899087311, -3.749999999999992006, 16.73437500000000000 ) ) ;
#58096=CARTESIAN_POINT ( 'NONE',  ( -2.694853999681181556, -10.10844685921792241, 18.93936829374151287 ) ) ;
#58102=CARTESIAN_POINT ( 'NONE',  ( -1.901340078031369618, -5.512252781505359245, 13.00186829374151465 ) ) ;
#58107=CARTESIAN_POINT ( 'NONE',  ( -2.749999999999998224, -7.500000000000015987, 16.34375000000000000 ) ) ;
#58197=CARTESIAN_POINT ( 'NONE',  ( -0.06109907496451398579, -10.25000000000000178, 16.28311829374151287 ) ) ;
#58306=CARTESIAN_POINT ( 'NONE',  ( 1.944543648263018731, -9.444543648262994751, 14.62500000000000000 ) ) ;
#58316=CARTESIAN_POINT ( 'NONE',  ( -2.749999999999997780, -7.561099074964547917, 22.34188170625849068 ) ) ;
#58325=CARTESIAN_POINT ( 'NONE',  ( -1.929879867024197893E-14, -3.750000000000000000, 17.90625000000000000 ) ) ;
#58361=CARTESIAN_POINT ( 'NONE',  ( 3.749999999999992006, -5.946699141100872943, 23.14062500000000000 ) ) ;
#58368=CARTESIAN_POINT ( 'NONE',  ( 2.320192649118979489E-14, -11.25000000000000000, 16.03125000000000000 ) ) ;
#58399=CARTESIAN_POINT ( 'NONE',  ( 2.694853999681214862, -10.10844685921789043, 20.62313170625849068 ) ) ;
#58410=CARTESIAN_POINT ( 'NONE',  ( 3.749999999999999556, -7.438900925035446754, 20.46688170625848713 ) ) ;
#58425=CARTESIAN_POINT ( 'NONE',  ( -1.492201783934593573, -3.724691934501250135, 13.07999329374151642 ) ) ;
#58503=CARTESIAN_POINT ( 'NONE',  ( 1.553300858899129944, -11.24999999999998934, 17.20312500000000000 ) ) ;
#58516=CARTESIAN_POINT ( 'NONE',  ( 3.750000000000000888, -7.499999999999978684, 16.96875000000000000 ) ) ;
#58530=CARTESIAN_POINT ( 'NONE',  ( -3.724691934501248802, -5.885600066136383646, 20.42374329374152353 ) ) ;
#58535=CARTESIAN_POINT ( 'NONE',  ( -1.944543648262992530, -9.444543648263016067, 26.18750000000000355 ) ) ;
#58542=CARTESIAN_POINT ( 'NONE',  ( -2.750000000000006217, -6.360912703474006946, 20.17187500000000000 ) ) ;
#58643=CARTESIAN_POINT ( 'NONE',  ( -0.06109907496451398579, -10.25000000000000178, 15.03311829374151287 ) ) ;
#58759=CARTESIAN_POINT ( 'NONE',  ( -1.944543648263014957, -5.555456351737005249, 14.00000000000000000 ) ) ;
#58761=CARTESIAN_POINT ( 'NONE',  ( 3.311681672511759267, -7.920257152778357401, 14.00000000000000888 ) ) ;
#58767=CARTESIAN_POINT ( 'NONE',  ( -1.139087296526025916, -4.750000000000006217, 16.57812500000000000 ) ) ;
#58775=CARTESIAN_POINT ( 'NONE',  ( 3.750000000000009770, -9.053300858899081760, 20.79687500000000000 ) ) ;
#58815=CARTESIAN_POINT ( 'NONE',  ( -2.651650429449535551, -10.15165042944956753, 19.93750000000000000 ) ) ;
#58821=CARTESIAN_POINT ( 'NONE',  ( 3.750000000000009770, -9.053300858899081760, 17.04687500000000000 ) ) ;
#58856=CARTESIAN_POINT ( 'NONE',  ( -3.749999999999996447, -7.561099074964554134, 23.59188170625849068 ) ) ;
#58869=CARTESIAN_POINT ( 'NONE',  ( -2.608446859217889546, -10.19485399968121264, 27.18563170625849068 ) ) ;
#58883=CARTESIAN_POINT ( 'NONE',  ( -2.724691934501246582, -6.299813628509474128, 24.17374329374151642 ) ) ;
#58962=CARTESIAN_POINT ( 'NONE',  ( -1.553300858899125059, -3.750000000000009326, 20.32812500000000000 ) ) ;
#58972=CARTESIAN_POINT ( 'NONE',  ( -2.651650429449535551, -10.15165042944956753, 18.68750000000000000 ) ) ;
#58989=CARTESIAN_POINT ( 'NONE',  ( -2.750000000000007105, -6.360912703474006946, 22.67187500000000355 ) ) ;
#58996=CARTESIAN_POINT ( 'NONE',  ( 2.750000000000008438, -8.639087296525996607, 18.29687500000000000 ) ) ;
#59091=CARTESIAN_POINT ( 'NONE',  ( -2.775308065498752086, -8.577988221561495763, 15.26749329374151465 ) ) ;
#59202=CARTESIAN_POINT ( 'NONE',  ( -1.987747218494660295, -5.598659921968651254, 26.24813170625849068 ) ) ;
#59211=CARTESIAN_POINT ( 'NONE',  ( -1.139087296526025916, -4.750000000000006217, 15.32812500000000355 ) ) ;
#59221=CARTESIAN_POINT ( 'NONE',  ( 3.749999999999992006, -5.946699141100872943, 21.89062500000000355 ) ) ;
#59264=CARTESIAN_POINT ( 'NONE',  ( 1.553300858899087311, -3.749999999999992006, 24.23437500000000355 ) ) ;
#59270=CARTESIAN_POINT ( 'NONE',  ( 3.749999999999992006, -5.946699141100872943, 14.39062500000000000 ) ) ;
#59302=CARTESIAN_POINT ( 'NONE',  ( 2.608446859217893099, -4.805146000318787358, 25.31063170625848713 ) ) ;
#59314=CARTESIAN_POINT ( 'NONE',  ( -1.200186371490556958, -4.775308065498765409, 15.07625670625849068 ) ) ;
#59327=CARTESIAN_POINT ( 'NONE',  ( 1.492201783934598236, -11.27530806549875031, 18.70499329374151287 ) ) ;
#59415=CARTESIAN_POINT ( 'NONE',  ( -2.651650429449535551, -10.15165042944956753, 23.68750000000000000 ) ) ;
#59423=CARTESIAN_POINT ( 'NONE',  ( 1.553300858899129944, -11.24999999999998934, 24.70312500000000000 ) ) ;
#59440=CARTESIAN_POINT ( 'NONE',  ( 2.724691934501250135, -8.700186371490531201, 14.79874329374151642 ) ) ;
#59447=CARTESIAN_POINT ( 'NONE',  ( -2.749999999999991562, -8.639087296526026805, 17.51562500000000000 ) ) ;
#59538=CARTESIAN_POINT ( 'NONE',  ( -1.987747218494638313, -9.401340078031370950, 16.43936829374151287 ) ) ;
#59646=CARTESIAN_POINT ( 'NONE',  ( 1.987747218494664292, -9.401340078031346081, 26.87313170625849423 ) ) ;
#59656=CARTESIAN_POINT ( 'NONE',  ( -1.987747218494660295, -5.598659921968651254, 27.49813170625849068 ) ) ;
#59666=CARTESIAN_POINT ( 'NONE',  ( -1.553300858899125059, -3.750000000000009326, 20.32812500000000000 ) ) ;
#59734=CARTESIAN_POINT ( 'NONE',  ( 0.02645256023170453746, -4.500116625257376768, 13.72411352175840626 ) ) ;
#59751=CARTESIAN_POINT ( 'NONE',  ( 0.06109907496455496689, -11.24999999999999822, 27.02938170625848358 ) ) ;
#59761=CARTESIAN_POINT ( 'NONE',  ( -2.724691934501232371, -8.700186371490559623, 16.01375670625849068 ) ) ;
#59774=CARTESIAN_POINT ( 'NONE',  ( -1.614399933863613468, -11.22469193450124969, 21.36124329374151642 ) ) ;
#59857=CARTESIAN_POINT ( 'NONE',  ( 3.749999999999992006, -5.946699141100872943, 23.14062500000000000 ) ) ;
#59865=CARTESIAN_POINT ( 'NONE',  ( -2.651650429449535551, -10.15165042944956753, 24.93750000000000000 ) ) ;
#59885=CARTESIAN_POINT ( 'NONE',  ( 1.077988221561497539, -10.27530806549875386, 14.95499329374151642 ) ) ;
#59889=CARTESIAN_POINT ( 'NONE',  ( 1.944543648263018731, -9.444543648262994751, 23.37500000000000000 ) ) ;
#59986=CARTESIAN_POINT ( 'NONE',  ( 1.077988221561497539, -10.27530806549875386, 16.20499329374151642 ) ) ;
#60088=CARTESIAN_POINT ( 'NONE',  ( -0.06109907496454585613, -4.750000000000000000, 26.40438170625848713 ) ) ;
#60100=CARTESIAN_POINT ( 'NONE',  ( -1.139087296526025916, -4.750000000000006217, 14.07812500000000178 ) ) ;
#60109=CARTESIAN_POINT ( 'NONE',  ( 2.320192649118979489E-14, -11.25000000000000000, 22.28125000000000355 ) ) ;
#60148=CARTESIAN_POINT ( 'NONE',  ( -2.651650429449535551, -10.15165042944956753, 26.18750000000000355 ) ) ;
#60155=CARTESIAN_POINT ( 'NONE',  ( 1.553300858899129722, -11.24999999999999112, 14.70312500000000355 ) ) ;
#60186=CARTESIAN_POINT ( 'NONE',  ( -1.200186371490556958, -4.775308065498765409, 15.07625670625849068 ) ) ;
#60200=CARTESIAN_POINT ( 'NONE',  ( 0.06109907496455496689, -11.24999999999999822, 25.77938170625848713 ) ) ;
#60208=CARTESIAN_POINT ( 'NONE',  ( 3.724691934501251023, -9.114399933863618131, 16.04874329374151287 ) ) ;
#60214=CARTESIAN_POINT ( 'NONE',  ( 3.750000000000001776, -7.561099074964511502, 19.72061829374151287 ) ) ;
#60298=CARTESIAN_POINT ( 'NONE',  ( -2.651650429449565305, -4.848349570550461785, 24.00000000000000000 ) ) ;
#60308=CARTESIAN_POINT ( 'NONE',  ( -3.749999999999997335, -7.500000000000021316, 25.09374999999999645 ) ) ;
#60323=CARTESIAN_POINT ( 'NONE',  ( 2.724691934501250135, -8.700186371490531201, 17.29874329374151642 ) ) ;
#60330=CARTESIAN_POINT ( 'NONE',  ( -1.409462824231155764E-14, -4.749999999999999112, 21.65625000000000355 ) ) ;
#60345=CIRCLE ( 'NONE', #21503, 0.4999999999999994449 ) ;
#60429=CARTESIAN_POINT ( 'NONE',  ( 0.06109907496451789238, -4.749999999999998224, 19.40811829374151287 ) ) ;
#60536=CARTESIAN_POINT ( 'NONE',  ( 2.750000000000001776, -7.499999999999984013, 19.46875000000000000 ) ) ;
#60545=CARTESIAN_POINT ( 'NONE',  ( 1.944543648263018731, -9.444543648262994751, 14.62500000000000000 ) ) ;
#60554=CARTESIAN_POINT ( 'NONE',  ( -3.749999999999997335, -7.500000000000021316, 20.09375000000000000 ) ) ;
#60599=CARTESIAN_POINT ( 'NONE',  ( 3.750000000000009770, -9.053300858899081760, 22.04687500000000000 ) ) ;
#60630=CARTESIAN_POINT ( 'NONE',  ( 1.492201783934554493, -3.724691934501233703, 23.98250670625849068 ) ) ;
#60642=CARTESIAN_POINT ( 'NONE',  ( -1.614399933863656544, -3.775308065498769405, 23.82625670625849068 ) ) ;
#60651=CARTESIAN_POINT ( 'NONE',  ( 3.775308065498752086, -6.007798216065404873, 18.39249329374151642 ) ) ;
#60657=CARTESIAN_POINT ( 'NONE',  ( 3.775308065498752086, -6.007798216065404873, 19.64249329374151642 ) ) ;
#60745=CARTESIAN_POINT ( 'NONE',  ( 1.553300858899129944, -11.24999999999998934, 22.20312500000000000 ) ) ;
#60753=CARTESIAN_POINT ( 'NONE',  ( -3.749999999999988454, -9.053300858899127945, 23.76562499999999645 ) ) ;
#60769=CARTESIAN_POINT ( 'NONE',  ( 2.775308065498755195, -6.422011778438505125, 14.64249329374151110 ) ) ;
#60776=CARTESIAN_POINT ( 'NONE',  ( 1.944543648262996083, -5.555456351736983045, 21.81250000000000000 ) ) ;
#60874=CARTESIAN_POINT ( 'NONE',  ( 2.724691934501250135, -8.700186371490531201, 21.04874329374151642 ) ) ;
#60896=SHAPE_REPRESENTATION_RELATIONSHIP ( 'NONE' , 'NONE' ,  #11000, #37432 ) ;
#60978=CARTESIAN_POINT ( 'NONE',  ( 1.944543648263018731, -9.444543648262994751, 18.37500000000000355 ) ) ;
#60989=CARTESIAN_POINT ( 'NONE',  ( 1.139087296525997273, -4.749999999999992895, 17.98437500000000000 ) ) ;
#60997=CARTESIAN_POINT ( 'NONE',  ( -2.651650429449565305, -4.848349570550461785, 24.00000000000000000 ) ) ;
#61047=CARTESIAN_POINT ( 'NONE',  ( -3.749999999999997335, -7.500000000000021316, 18.84375000000000000 ) ) ;
#61077=CARTESIAN_POINT ( 'NONE',  ( -0.06109907496454585613, -4.750000000000000000, 18.90438170625848713 ) ) ;
#61089=CARTESIAN_POINT ( 'NONE',  ( -1.200186371490556958, -4.775308065498765409, 20.07625670625849068 ) ) ;
#61096=CARTESIAN_POINT ( 'NONE',  ( 2.608446859217924629, -10.19485399968118422, 24.87686829374151642 ) ) ;
#61103=CARTESIAN_POINT ( 'NONE',  ( 1.492201783934598236, -11.27530806549875031, 19.95499329374151642 ) ) ;
#61179=CARTESIAN_POINT ( 'NONE',  ( 3.775308065498768517, -8.992201783934554271, 16.79500670625849068 ) ) ;
#61187=CARTESIAN_POINT ( 'NONE',  ( -1.553300858899081538, -11.25000000000000711, 26.10937500000001066 ) ) ;
#61202=CARTESIAN_POINT ( 'NONE',  ( -2.724691934501246582, -6.299813628509474128, 17.92374329374151287 ) ) ;
#61211=CARTESIAN_POINT ( 'NONE',  ( -1.944543648262992530, -9.444543648263016067, 23.68750000000000000 ) ) ;
#61301=CARTESIAN_POINT ( 'NONE',  ( -1.200186371490524317, -10.22469193450124791, 21.36124329374151642 ) ) ;
#61412=CARTESIAN_POINT ( 'NONE',  ( -1.409462824231155764E-14, -4.749999999999999112, 20.40625000000000000 ) ) ;
#61425=CARTESIAN_POINT ( 'NONE',  ( 1.139087296526029469, -10.24999999999999467, 19.70312500000000355 ) ) ;
#61485=CARTESIAN_POINT ( 'NONE',  ( 3.749999999999992006, -5.946699141100872943, 18.14062500000000355 ) ) ;
#61514=CARTESIAN_POINT ( 'NONE',  ( 1.077988221561464899, -4.724691934501233703, 16.48250670625849423 ) ) ;
#61526=CARTESIAN_POINT ( 'NONE',  ( 2.750000000000001332, -7.438900925035452083, 20.46688170625848713 ) ) ;
#61534=CARTESIAN_POINT ( 'NONE',  ( 0.06109907496451268821, -3.749999999999999556, 20.65811829374151287 ) ) ;
#61541=CARTESIAN_POINT ( 'NONE',  ( -2.608446859217920633, -4.805146000318815780, 25.50186829374151287 ) ) ;
#61625=CARTESIAN_POINT ( 'NONE',  ( -1.492201783934549164, -11.27530806549876807, 15.85750670625849068 ) ) ;
#61634=CARTESIAN_POINT ( 'NONE',  ( 3.750000000000000888, -7.499999999999978684, 25.71875000000000000 ) ) ;
#61649=CARTESIAN_POINT ( 'NONE',  ( -1.077988221561493543, -4.724691934501247914, 21.82999329374151642 ) ) ;
#61655=CARTESIAN_POINT ( 'NONE',  ( 2.750000000000001776, -7.499999999999984013, 24.46875000000000000 ) ) ;
#61747=CARTESIAN_POINT ( 'NONE',  ( -1.901340078031369618, -5.512252781505359245, 23.00186829374151287 ) ) ;
#61808=CARTESIAN_POINT ( 'NONE',  ( 2.651650429449569302, -10.15165042944953733, 25.87500000000000355 ) ) ;
#61856=CARTESIAN_POINT ( 'NONE',  ( 1.944543648262996083, -5.555456351736983045, 19.31250000000000000 ) ) ;
#61864=CARTESIAN_POINT ( 'NONE',  ( -1.944543648263014957, -5.555456351737005249, 19.00000000000000000 ) ) ;
#61873=CARTESIAN_POINT ( 'NONE',  ( -3.750000000000008438, -5.946699141100917352, 26.42187500000000000 ) ) ;
#61925=CARTESIAN_POINT ( 'NONE',  ( 2.651650429449539104, -4.848349570550432475, 20.56250000000000000 ) ) ;
#61929=VERTEX_POINT ( 'NONE', #4943 ) ;
#61959=CARTESIAN_POINT ( 'NONE',  ( -1.200186371490556958, -4.775308065498765409, 18.82625670625848713 ) ) ;
#61972=CARTESIAN_POINT ( 'NONE',  ( 1.901340078031349856, -5.512252781505337929, 17.81063170625849068 ) ) ;
#61981=CARTESIAN_POINT ( 'NONE',  ( 3.750000000000001776, -7.561099074964511502, 20.97061829374151642 ) ) ;
#61988=CARTESIAN_POINT ( 'NONE',  ( -3.749999999999997780, -7.438900925035489387, 22.84561829374151642 ) ) ;
#62072=CARTESIAN_POINT ( 'NONE',  ( 3.724691934501232815, -5.885600066136343678, 15.38875670625848890 ) ) ;
#62082=CARTESIAN_POINT ( 'NONE',  ( -1.492201783934549164, -11.27530806549876807, 18.35750670625849068 ) ) ;
#62099=CARTESIAN_POINT ( 'NONE',  ( -1.200186371490524317, -10.22469193450124791, 20.11124329374151642 ) ) ;
#62148=ORIENTED_EDGE ( 'NONE', *, *, #55896, .F. ) ;
#62186=CARTESIAN_POINT ( 'NONE',  ( -3.749999999999988454, -9.053300858899127945, 15.01562500000000178 ) ) ;
#62202=CARTESIAN_POINT ( 'NONE',  ( -1.987747218494638313, -9.401340078031370950, 20.18936829374151287 ) ) ;
#62251=CARTESIAN_POINT ( 'NONE',  ( -1.553300858899125059, -3.750000000000009326, 25.32812500000000711 ) ) ;
#62301=CARTESIAN_POINT ( 'NONE',  ( 1.139087296525997273, -4.749999999999992895, 20.48437500000000000 ) ) ;
#62365=CARTESIAN_POINT ( 'NONE',  ( 3.750000000000000888, -7.499999999999978684, 18.21875000000000000 ) ) ;
#62394=CARTESIAN_POINT ( 'NONE',  ( 0.06109907496454976272, -10.25000000000000000, 19.52938170625848713 ) ) ;
#62406=CARTESIAN_POINT ( 'NONE',  ( -2.724691934501232371, -8.700186371490559623, 18.51375670625849068 ) ) ;
#62414=CARTESIAN_POINT ( 'NONE',  ( -2.694853999681181556, -10.10844685921792241, 23.93936829374151642 ) ) ;
#62420=CARTESIAN_POINT ( 'NONE',  ( -2.608446859217920633, -4.805146000318815780, 21.75186829374151287 ) ) ;
#62502=CARTESIAN_POINT ( 'NONE',  ( -0.06109907496455085213, -3.750000000000000888, 15.15438170625848890 ) ) ;
#62512=CARTESIAN_POINT ( 'NONE',  ( 1.614399933863660985, -11.22469193450123193, 15.70125670625848890 ) ) ;
#62527=CARTESIAN_POINT ( 'NONE',  ( 1.077988221561497539, -10.27530806549875386, 22.45499329374151287 ) ) ;
#62635=CARTESIAN_POINT ( 'NONE',  ( 3.724691934501251023, -9.114399933863618131, 13.54874329374151465 ) ) ;
#62740=CARTESIAN_POINT ( 'NONE',  ( -2.750000000000007105, -6.360912703474006946, 22.67187500000000355 ) ) ;
#62763=CARTESIAN_POINT ( 'NONE',  ( 0.000000000000000000, 0.000000000000000000, 0.000000000000000000 ) ) ;
#62832=CARTESIAN_POINT ( 'NONE',  ( -1.200186371490556958, -4.775308065498765409, 22.57625670625848713 ) ) ;
#62844=CARTESIAN_POINT ( 'NONE',  ( -1.200186371490556958, -4.775308065498765409, 16.32625670625849068 ) ) ;
#62852=CARTESIAN_POINT ( 'NONE',  ( 2.694853999681185108, -4.891553140782077591, 24.56436829374151287 ) ) ;
#62859=CARTESIAN_POINT ( 'NONE',  ( 1.614399933863618797, -3.775308065498751198, 23.23624329374151642 ) ) ;
#62942=CARTESIAN_POINT ( 'NONE',  ( 3.750000000000009770, -9.053300858899081760, 24.54687500000000000 ) ) ;
#62950=CARTESIAN_POINT ( 'NONE',  ( -1.553300858899125059, -3.750000000000009326, 25.32812500000000711 ) ) ;
#62967=CARTESIAN_POINT ( 'NONE',  ( 1.901340078031373171, -9.487747218494639867, 21.12686829374151287 ) ) ;
#63077=CARTESIAN_POINT ( 'NONE',  ( -1.200186371490524317, -10.22469193450124791, 23.86124329374151998 ) ) ;
#63086=CARTESIAN_POINT ( 'NONE',  ( 2.750000000000008438, -8.639087296525996607, 14.54687500000000000 ) ) ;
#63188=CARTESIAN_POINT ( 'NONE',  ( -2.750000000000007105, -6.360912703474006946, 25.17187500000000000 ) ) ;
#63261=CARTESIAN_POINT ( 'NONE',  ( 2.651650429449539104, -4.848349570550432475, 24.31250000000000000 ) ) ;
#63288=CARTESIAN_POINT ( 'NONE',  ( -1.944543648263014957, -5.555456351737005249, 14.00000000000000000 ) ) ;
#63291=CARTESIAN_POINT ( 'NONE',  ( -2.775308065498764964, -6.422011778438537988, 22.42000670625849068 ) ) ;
#63295=ORIENTED_EDGE ( 'NONE', *, *, #11973, .F. ) ;
#63304=CARTESIAN_POINT ( 'NONE',  ( -2.775308065498764964, -6.422011778438537988, 21.17000670625848713 ) ) ;
#63314=CARTESIAN_POINT ( 'NONE',  ( 1.553300858899129944, -11.24999999999998934, 18.45312500000000355 ) ) ;
#63320=CARTESIAN_POINT ( 'NONE',  ( -3.724691934501248802, -5.885600066136383646, 24.17374329374151642 ) ) ;
#63397=CARTESIAN_POINT ( 'NONE',  ( 1.614399933863660985, -11.22469193450123193, 18.20125670625849068 ) ) ;
#63406=CARTESIAN_POINT ( 'NONE',  ( 1.492201783934554493, -3.724691934501233703, 18.98250670625849068 ) ) ;
#63422=CARTESIAN_POINT ( 'NONE',  ( 2.750000000000002665, -7.561099074964516831, 22.22061829374151287 ) ) ;
#63502=CARTESIAN_POINT ( 'NONE',  ( 2.320192649118979489E-14, -11.25000000000000000, 18.53125000000000000 ) ) ;
#63513=CARTESIAN_POINT ( 'NONE',  ( 3.749999999999992006, -5.946699141100872943, 14.39062500000000178 ) ) ;
#63526=CARTESIAN_POINT ( 'NONE',  ( 0.06109907496451268821, -3.749999999999999556, 14.40811829374151110 ) ) ;
#63530=CARTESIAN_POINT ( 'NONE',  ( -1.139087296526025916, -4.750000000000006217, 17.82812500000000000 ) ) ;
#63535=CARTESIAN_POINT ( 'NONE',  ( 2.750000000000001776, -7.499999999999984013, 15.71875000000000000 ) ) ;
#63635=CARTESIAN_POINT ( 'NONE',  ( 2.749999999999995115, -6.360912703473971419, 23.14062500000000000 ) ) ;
#63702=CARTESIAN_POINT ( 'NONE',  ( 3.750000000000000888, -7.499999999999978684, 23.21875000000000000 ) ) ;
#63734=CARTESIAN_POINT ( 'NONE',  ( -1.200186371490556958, -4.775308065498765409, 23.82625670625849068 ) ) ;
#63738=CARTESIAN_POINT ( 'NONE',  ( 3.446590374638324406, -6.824229032706653264, 14.00000000000008349 ) ) ;
#63747=CARTESIAN_POINT ( 'NONE',  ( -1.987747218494660295, -5.598659921968651254, 23.74813170625849068 ) ) ;
#63755=CARTESIAN_POINT ( 'NONE',  ( 3.749999999999992006, -5.946699141100872943, 14.39062500000000178 ) ) ;
#63759=CARTESIAN_POINT ( 'NONE',  ( -2.651650429449565305, -4.848349570550461785, 16.50000000000000000 ) ) ;
#63799=CARTESIAN_POINT ( 'NONE',  ( 3.749999999999992006, -5.946699141100872943, 19.39062500000000711 ) ) ;
#63844=CARTESIAN_POINT ( 'NONE',  ( 3.724691934501232815, -5.885600066136343678, 17.88875670625848713 ) ) ;
#63852=CARTESIAN_POINT ( 'NONE',  ( -1.492201783934549164, -11.27530806549876807, 23.35750670625849423 ) ) ;
#63866=CARTESIAN_POINT ( 'NONE',  ( -1.614399933863613468, -11.22469193450124969, 15.11124329374151287 ) ) ;
#63939=CARTESIAN_POINT ( 'NONE',  ( 3.750000000000000888, -7.499999999999978684, 18.21875000000000000 ) ) ;
#63950=CARTESIAN_POINT ( 'NONE',  ( -1.553300858899081538, -11.25000000000000711, 16.10937500000000355 ) ) ;
#63963=CARTESIAN_POINT ( 'NONE',  ( 3.724691934501251023, -9.114399933863618131, 14.79874329374151642 ) ) ;
#63967=CARTESIAN_POINT ( 'NONE',  ( 2.750000000000008438, -8.639087296525996607, 23.29687500000000000 ) ) ;
#63971=CARTESIAN_POINT ( 'NONE',  ( 1.139087296525997051, -4.749999999999992895, 15.48437499999999822 ) ) ;
#64071=CARTESIAN_POINT ( 'NONE',  ( -1.139087296525992166, -10.25000000000000533, 24.85937500000001421 ) ) ;
#64168=CARTESIAN_POINT ( 'NONE',  ( -2.749999999999997780, -7.561099074964547917, 23.59188170625849068 ) ) ;
#64178=CARTESIAN_POINT ( 'NONE',  ( 2.775308065498768517, -8.577988221561467341, 21.79500670625849068 ) ) ;
#64185=CARTESIAN_POINT ( 'NONE',  ( 1.553300858899129944, -11.24999999999998934, 17.20312500000000000 ) ) ;
#64190=CARTESIAN_POINT ( 'NONE',  ( 2.320192649118979489E-14, -11.25000000000000000, 17.28125000000000000 ) ) ;
#64230=CARTESIAN_POINT ( 'NONE',  ( 2.320192649118979489E-14, -11.25000000000000000, 22.28125000000000355 ) ) ;
#64274=CARTESIAN_POINT ( 'NONE',  ( -0.06109907496455085213, -3.750000000000000888, 20.15438170625849068 ) ) ;
#64281=CARTESIAN_POINT ( 'NONE',  ( -2.694853999681210865, -4.891553140782108677, 22.49813170625848713 ) ) ;
#64297=CARTESIAN_POINT ( 'NONE',  ( 1.077988221561497539, -10.27530806549875386, 24.95499329374151287 ) ) ;
#64376=CARTESIAN_POINT ( 'NONE',  ( 1.553300858899129944, -11.24999999999998934, 18.45312500000000355 ) ) ;
#64387=CARTESIAN_POINT ( 'NONE',  ( 2.651650429449569302, -10.15165042944953733, 19.62500000000000000 ) ) ;
#64400=CARTESIAN_POINT ( 'NONE',  ( 0.06109907496451268821, -3.749999999999999556, 18.15811829374151642 ) ) ;
#64404=CARTESIAN_POINT ( 'NONE',  ( 2.750000000000001776, -7.499999999999984013, 24.46875000000000000 ) ) ;
#64409=CARTESIAN_POINT ( 'NONE',  ( 2.749999999999995115, -6.360912703473971419, 15.64062500000000178 ) ) ;
#64498=CARTESIAN_POINT ( 'NONE',  ( -1.139087296525992166, -10.25000000000000533, 26.10937500000001066 ) ) ;
#64575=CARTESIAN_POINT ( 'NONE',  ( 1.553300858899086867, -3.749999999999992006, 25.48437500000000000 ) ) ;
#64610=CARTESIAN_POINT ( 'NONE',  ( -1.077988221561460236, -10.27530806549876452, 20.85750670625849068 ) ) ;
#64612=CARTESIAN_POINT ( 'NONE',  ( 3.460919881479461502, -7.042993046541733193, 14.00000000000001421 ) ) ;
#64620=CARTESIAN_POINT ( 'NONE',  ( 0.06109907496454976272, -10.25000000000000000, 25.77938170625848713 ) ) ;
#64630=CARTESIAN_POINT ( 'NONE',  ( -1.553300858899125059, -3.750000000000009326, 16.57812500000000000 ) ) ;
#64635=CARTESIAN_POINT ( 'NONE',  ( 3.750000000000000888, -7.499999999999978684, 16.96875000000000000 ) ) ;
#64676=CARTESIAN_POINT ( 'NONE',  ( 2.320192649118979489E-14, -11.25000000000000000, 23.53125000000000000 ) ) ;
#64695=AXIS2_PLACEMENT_3D ( 'NONE', #39796, #53740, #81226 ) ;
#64718=CARTESIAN_POINT ( 'NONE',  ( -0.06109907496455085213, -3.750000000000000888, 21.40438170625849068 ) ) ;
#64726=CARTESIAN_POINT ( 'NONE',  ( 0.06109907496455496689, -11.24999999999999822, 20.77938170625848713 ) ) ;
#64740=CARTESIAN_POINT ( 'NONE',  ( 1.492201783934598236, -11.27530806549875031, 16.20499329374151642 ) ) ;
#64818=CARTESIAN_POINT ( 'NONE',  ( 3.750000000000009770, -9.053300858899081760, 14.54687500000000178 ) ) ;
#64829=CARTESIAN_POINT ( 'NONE',  ( -2.651650429449565305, -4.848349570550461785, 20.25000000000000000 ) ) ;
#64846=CARTESIAN_POINT ( 'NONE',  ( -2.608446859217920633, -4.805146000318815780, 18.00186829374151287 ) ) ;
#64852=CARTESIAN_POINT ( 'NONE',  ( 2.749999999999995115, -6.360912703473971419, 25.64062500000000000 ) ) ;
#64856=CARTESIAN_POINT ( 'NONE',  ( 2.750000000000008438, -8.639087296525996607, 19.54687500000000000 ) ) ;
#64953=CARTESIAN_POINT ( 'NONE',  ( -1.987747218494638313, -9.401340078031370950, 13.93936829374151465 ) ) ;
#65057=CARTESIAN_POINT ( 'NONE',  ( 2.750000000000001776, -7.499999999999984013, 14.46875000000000000 ) ) ;
#65069=CARTESIAN_POINT ( 'NONE',  ( 1.987747218494664292, -9.401340078031346081, 23.12313170625848713 ) ) ;
#65077=CARTESIAN_POINT ( 'NONE',  ( 3.750000000000000888, -7.499999999999978684, 16.96875000000000000 ) ) ;
#65081=CARTESIAN_POINT ( 'NONE',  ( 2.651650429449539104, -4.848349570550432475, 15.56250000000000000 ) ) ;
#65120=CARTESIAN_POINT ( 'NONE',  ( 3.750000000000009770, -9.053300858899081760, 20.79687500000000000 ) ) ;
#65129=CARTESIAN_POINT ( 'NONE',  ( 2.651650429449539104, -4.848349570550432475, 15.56250000000000000 ) ) ;
#65164=CARTESIAN_POINT ( 'NONE',  ( -3.775308065498766297, -6.007798216065450170, 22.42000670625849068 ) ) ;
#65175=CARTESIAN_POINT ( 'NONE',  ( 3.724691934501232815, -5.885600066136343678, 21.63875670625848713 ) ) ;
#65189=CARTESIAN_POINT ( 'NONE',  ( -2.775308065498752086, -8.577988221561495763, 24.01749329374151287 ) ) ;
#65271=CARTESIAN_POINT ( 'NONE',  ( 3.750000000000009770, -9.053300858899081760, 15.79687500000000178 ) ) ;
#65283=CARTESIAN_POINT ( 'NONE',  ( -1.553300858899125059, -3.750000000000009326, 16.57812500000000000 ) ) ;
#65298=CARTESIAN_POINT ( 'NONE',  ( -1.614399933863613468, -11.22469193450124969, 18.86124329374151287 ) ) ;
#65303=CARTESIAN_POINT ( 'NONE',  ( 1.139087296526029469, -10.24999999999999467, 25.95312500000000000 ) ) ;
#65308=CARTESIAN_POINT ( 'NONE',  ( 2.749999999999995115, -6.360912703473971419, 20.64062500000000000 ) ) ;
#65405=CARTESIAN_POINT ( 'NONE',  ( -1.901340078031369618, -5.512252781505359245, 14.25186829374151465 ) ) ;
#65512=CARTESIAN_POINT ( 'NONE',  ( -2.749999999999997780, -7.561099074964547917, 26.09188170625848358 ) ) ;
#65521=CARTESIAN_POINT ( 'NONE',  ( 2.750000000000008438, -8.639087296525996607, 17.04687500000000000 ) ) ;
#65529=CARTESIAN_POINT ( 'NONE',  ( -3.749999999999988454, -9.053300858899127945, 20.01562500000000355 ) ) ;
#65568=CARTESIAN_POINT ( 'NONE',  ( -1.553300858899125059, -3.750000000000009326, 20.32812500000000000 ) ) ;
#65575=CARTESIAN_POINT ( 'NONE',  ( 1.553300858899129722, -11.24999999999999112, 15.95312499999999822 ) ) ;
#65604=CARTESIAN_POINT ( 'NONE',  ( 3.749999999999999556, -7.438900925035446754, 24.21688170625849068 ) ) ;
#65613=CARTESIAN_POINT ( 'NONE',  ( -0.06109907496454585613, -4.750000000000000000, 15.15438170625848890 ) ) ;
#65626=CARTESIAN_POINT ( 'NONE',  ( -2.749999999999999112, -7.438900925035484057, 24.09561829374151287 ) ) ;
#65712=CARTESIAN_POINT ( 'NONE',  ( -2.651650429449565305, -4.848349570550461785, 20.25000000000000000 ) ) ;
#65723=CARTESIAN_POINT ( 'NONE',  ( -1.553300858899081538, -11.25000000000000711, 18.60937500000000355 ) ) ;
#65740=CARTESIAN_POINT ( 'NONE',  ( -1.139087296526025916, -4.750000000000006217, 24.07812500000000355 ) ) ;
#65747=CARTESIAN_POINT ( 'NONE',  ( -2.750000000000006217, -6.360912703474006946, 18.92187500000000000 ) ) ;
#65840=CARTESIAN_POINT ( 'NONE',  ( 1.901340078031373171, -9.487747218494639867, 13.62686829374151642 ) ) ;
#65873=DIRECTION ( 'NONE',  ( -0.7071067811865510144, 0.7071067811865440200, 0.000000000000000000 ) ) ;
#65954=CARTESIAN_POINT ( 'NONE',  ( -1.409462824231155764E-14, -4.749999999999999112, 14.15625000000000000 ) ) ;
#65963=CARTESIAN_POINT ( 'NONE',  ( 0.06109907496454976272, -10.25000000000000000, 27.02938170625848358 ) ) ;
#65972=CARTESIAN_POINT ( 'NONE',  ( 2.651650429449539104, -4.848349570550432475, 19.31250000000000000 ) ) ;
#66019=CARTESIAN_POINT ( 'NONE',  ( 2.651650429449539104, -4.848349570550432475, 14.31250000000000000 ) ) ;
#66052=CARTESIAN_POINT ( 'NONE',  ( 2.694853999681214862, -10.10844685921789043, 24.37313170625848713 ) ) ;
#66062=CARTESIAN_POINT ( 'NONE',  ( -3.775308065498766297, -6.007798216065450170, 26.17000670625849068 ) ) ;
#66078=CARTESIAN_POINT ( 'NONE',  ( 2.694853999681185108, -4.891553140782077591, 17.06436829374151287 ) ) ;
#66135=EDGE_CURVE ( 'NONE', #25338, #58074, #42057, .T. ) ;
#66162=CARTESIAN_POINT ( 'NONE',  ( -2.651650429449535551, -10.15165042944956753, 21.18750000000000000 ) ) ;
#66170=CARTESIAN_POINT ( 'NONE',  ( 3.750000000000009770, -9.053300858899081760, 24.54687500000000000 ) ) ;
#66189=CARTESIAN_POINT ( 'NONE',  ( -2.775308065498752086, -8.577988221561495763, 15.26749329374151465 ) ) ;
#66198=CARTESIAN_POINT ( 'NONE',  ( 2.750000000000001776, -7.499999999999984013, 16.96875000000000000 ) ) ;
#66297=CARTESIAN_POINT ( 'NONE',  ( 2.750000000000002665, -7.561099074964516831, 14.72061829374151465 ) ) ;
#66410=CARTESIAN_POINT ( 'NONE',  ( 1.139087296526029469, -10.24999999999999467, 15.95312500000000000 ) ) ;
#66420=CARTESIAN_POINT ( 'NONE',  ( -2.749999999999998224, -7.500000000000015987, 16.34375000000000000 ) ) ;
#66430=CARTESIAN_POINT ( 'NONE',  ( -3.749999999999988454, -9.053300858899127945, 23.76562499999999645 ) ) ;
#66482=CARTESIAN_POINT ( 'NONE',  ( -1.553300858899081760, -11.25000000000000888, 16.10937500000000355 ) ) ;
#66512=CARTESIAN_POINT ( 'NONE',  ( 1.614399933863660985, -11.22469193450123193, 24.45125670625849423 ) ) ;
#66525=CARTESIAN_POINT ( 'NONE',  ( -1.901340078031346525, -9.487747218494661183, 15.93563170625849068 ) ) ;
#66540=CARTESIAN_POINT ( 'NONE',  ( 3.724691934501251023, -9.114399933863618131, 21.04874329374151642 ) ) ;
#66623=CARTESIAN_POINT ( 'NONE',  ( 2.320192649118979489E-14, -11.25000000000000000, 21.03125000000000000 ) ) ;
#66631=CARTESIAN_POINT ( 'NONE',  ( -1.553300858899081538, -11.25000000000000711, 22.35937500000000711 ) ) ;
#66647=CARTESIAN_POINT ( 'NONE',  ( -1.901340078031369618, -5.512252781505359245, 14.25186829374151465 ) ) ;
#66654=CARTESIAN_POINT ( 'NONE',  ( 1.139087296525997051, -4.749999999999992895, 19.23437500000000000 ) ) ;
#66745=CARTESIAN_POINT ( 'NONE',  ( -1.987747218494638313, -9.401340078031370950, 15.18936829374151465 ) ) ;
#66858=CARTESIAN_POINT ( 'NONE',  ( 2.775308065498768517, -8.577988221561467341, 26.79500670625849423 ) ) ;
#66867=CARTESIAN_POINT ( 'NONE',  ( 1.139087296525997273, -4.749999999999992895, 15.48437500000000178 ) ) ;
#66877=CARTESIAN_POINT ( 'NONE',  ( 2.651650429449539104, -4.848349570550432475, 20.56250000000000000 ) ) ;
#66918=CARTESIAN_POINT ( 'NONE',  ( -1.929879867024197893E-14, -3.750000000000000000, 24.15625000000000000 ) ) ;
#66957=CARTESIAN_POINT ( 'NONE',  ( 1.492201783934554493, -3.724691934501233703, 26.48250670625848713 ) ) ;
#66971=CARTESIAN_POINT ( 'NONE',  ( -2.608446859217889546, -10.19485399968121264, 24.68563170625849068 ) ) ;
#66979=CARTESIAN_POINT ( 'NONE',  ( -3.775308065498748977, -8.992201783934593351, 16.51749329374151642 ) ) ;
#66987=CARTESIAN_POINT ( 'NONE',  ( 1.614399933863618797, -3.775308065498751198, 18.23624329374151642 ) ) ;
#67018=ORIENTED_EDGE ( 'NONE', *, *, #55896, .T. ) ;
#67067=CARTESIAN_POINT ( 'NONE',  ( 1.553300858899129944, -11.24999999999998934, 19.70312500000000355 ) ) ;
#67077=CARTESIAN_POINT ( 'NONE',  ( 3.749999999999992006, -5.946699141100872943, 24.39062500000000000 ) ) ;
#67094=CARTESIAN_POINT ( 'NONE',  ( -1.077988221561493543, -4.724691934501247914, 15.57999329374151110 ) ) ;
#67101=CARTESIAN_POINT ( 'NONE',  ( 1.944543648263018731, -9.444543648262994751, 24.62500000000000000 ) ) ;
#67133=ORIENTED_EDGE ( 'NONE', *, *, #11973, .T. ) ;
#67200=CARTESIAN_POINT ( 'NONE',  ( 2.750000000000002665, -7.561099074964516831, 20.97061829374151642 ) ) ;
#67237=ORIENTED_EDGE ( 'NONE', *, *, #66135, .T. ) ;
#67283=CARTESIAN_POINT ( 'NONE',  ( 2.651650429449539104, -4.848349570550432475, 14.31250000000000000 ) ) ;
#67304=CARTESIAN_POINT ( 'NONE',  ( 2.749999999999995115, -6.360912703473971419, 18.14062500000000711 ) ) ;
#67312=CARTESIAN_POINT ( 'NONE',  ( -1.139087296525992166, -10.25000000000000533, 16.10937500000000355 ) ) ;
#67320=CARTESIAN_POINT ( 'NONE',  ( 2.651650429449569302, -10.15165042944953733, 23.37500000000000000 ) ) ;
#67368=CARTESIAN_POINT ( 'NONE',  ( 1.553300858899129722, -11.24999999999999112, 22.20312500000000000 ) ) ;
#67398=CARTESIAN_POINT ( 'NONE',  ( 3.749999999999999556, -7.438900925035446754, 25.46688170625849423 ) ) ;
#67411=CARTESIAN_POINT ( 'NONE',  ( 3.749999999999999556, -7.438900925035446754, 24.21688170625849068 ) ) ;
#67418=CARTESIAN_POINT ( 'NONE',  ( -2.694853999681181556, -10.10844685921792241, 16.43936829374151287 ) ) ;
#67425=CARTESIAN_POINT ( 'NONE',  ( -3.775308065498748977, -8.992201783934593351, 17.76749329374151287 ) ) ;
#67513=CARTESIAN_POINT ( 'NONE',  ( 3.750000000000009770, -9.053300858899081760, 19.54687499999999645 ) ) ;
#67521=CARTESIAN_POINT ( 'NONE',  ( 2.651650429449539104, -4.848349570550432475, 23.06250000000000000 ) ) ;
#67536=CARTESIAN_POINT ( 'NONE',  ( -1.901340078031369618, -5.512252781505359245, 16.75186829374151287 ) ) ;
#67543=CARTESIAN_POINT ( 'NONE',  ( 1.799775606325937360E-14, -10.25000000000000000, 23.53125000000000000 ) ) ;
#67641=CARTESIAN_POINT ( 'NONE',  ( -0.06109907496451398579, -10.25000000000000178, 20.03311829374151287 ) ) ;
#67744=CARTESIAN_POINT ( 'NONE',  ( -1.139087296525992166, -10.25000000000000533, 19.85937500000000355 ) ) ;
#67754=CARTESIAN_POINT ( 'NONE',  ( -2.750000000000007105, -6.360912703474006946, 17.67187500000000355 ) ) ;
#67811=CARTESIAN_POINT ( 'NONE',  ( 1.553300858899086867, -3.749999999999992006, 20.48437500000000000 ) ) ;
#67841=CARTESIAN_POINT ( 'NONE',  ( -2.724691934501232371, -8.700186371490559623, 16.01375670625849068 ) ) ;
#67853=CARTESIAN_POINT ( 'NONE',  ( -1.901340078031346525, -9.487747218494661183, 19.68563170625849068 ) ) ;
#67860=CARTESIAN_POINT ( 'NONE',  ( 2.694853999681185108, -4.891553140782077591, 20.81436829374151287 ) ) ;
#67867=CARTESIAN_POINT ( 'NONE',  ( -2.694853999681181556, -10.10844685921792241, 18.93936829374151287 ) ) ;
#67956=CARTESIAN_POINT ( 'NONE',  ( 1.553300858899087311, -3.749999999999992006, 25.48437500000000000 ) ) ;
#67965=CARTESIAN_POINT ( 'NONE',  ( -2.651650429449565305, -4.848349570550461785, 21.50000000000000000 ) ) ;
#67983=CARTESIAN_POINT ( 'NONE',  ( -2.749999999999999112, -7.438900925035484057, 17.84561829374150932 ) ) ;
#67991=CARTESIAN_POINT ( 'NONE',  ( 1.139087296526029469, -10.24999999999999289, 23.45312500000000000 ) ) ;
#68018=EDGE_LOOP ( 'NONE', ( #67018, #11850, #38386, #47313 ) ) ;
#68087=CARTESIAN_POINT ( 'NONE',  ( 1.077988221561497539, -10.27530806549875386, 22.45499329374151287 ) ) ;
#68188=CARTESIAN_POINT ( 'NONE',  ( -2.750000000000007105, -6.360912703474006946, 20.17187500000000000 ) ) ;
#68199=CARTESIAN_POINT ( 'NONE',  ( -1.139087296525992166, -10.25000000000000533, 21.10937500000000711 ) ) ;
#68206=CARTESIAN_POINT ( 'NONE',  ( -3.750000000000008438, -5.946699141100917352, 23.92187500000000355 ) ) ;
#68254=CARTESIAN_POINT ( 'NONE',  ( -3.750000000000007550, -5.946699141100917352, 21.42187500000000000 ) ) ;
#68281=CARTESIAN_POINT ( 'NONE',  ( -2.775308065498764964, -6.422011778438537988, 17.42000670625848713 ) ) ;
#68284=CARTESIAN_POINT ( 'NONE',  ( 0.5140118631390264703, -3.794621124119502031, 14.00000000000000178 ) ) ;
#68294=CARTESIAN_POINT ( 'NONE',  ( -2.749999999999997780, -7.561099074964547917, 18.59188170625849068 ) ) ;
#68302=CARTESIAN_POINT ( 'NONE',  ( 1.614399933863618797, -3.775308065498751198, 23.23624329374151642 ) ) ;
#68309=CARTESIAN_POINT ( 'NONE',  ( -1.492201783934593573, -3.724691934501250135, 23.07999329374151998 ) ) ;
#68388=CARTESIAN_POINT ( 'NONE',  ( -2.694853999681210865, -4.891553140782108677, 16.24813170625848713 ) ) ;
#68398=CARTESIAN_POINT ( 'NONE',  ( -3.749999999999996447, -7.561099074964554134, 17.34188170625849068 ) ) ;
#68414=CARTESIAN_POINT ( 'NONE',  ( 1.077988221561497539, -10.27530806549875386, 19.95499329374151642 ) ) ;
#68421=CARTESIAN_POINT ( 'NONE',  ( -1.139087296526025250, -4.750000000000006217, 24.07812500000000711 ) ) ;
#68515=CARTESIAN_POINT ( 'NONE',  ( -1.077988221561493543, -4.724691934501247914, 21.82999329374151642 ) ) ;
#68624=CARTESIAN_POINT ( 'NONE',  ( -2.749999999999998224, -7.500000000000015987, 18.84375000000000000 ) ) ;
#68634=CARTESIAN_POINT ( 'NONE',  ( -1.944543648262992530, -9.444543648263016067, 22.43750000000000000 ) ) ;
#68641=CARTESIAN_POINT ( 'NONE',  ( 3.750000000000000888, -7.499999999999978684, 24.46875000000000000 ) ) ;
#68691=CARTESIAN_POINT ( 'NONE',  ( -1.553300858899125059, -3.750000000000009326, 21.57812500000000355 ) ) ;
#68725=CARTESIAN_POINT ( 'NONE',  ( -1.077988221561460236, -10.27530806549876452, 15.85750670625849068 ) ) ;
#68737=CARTESIAN_POINT ( 'NONE',  ( -2.749999999999997780, -7.561099074964547917, 19.84188170625848713 ) ) ;
#68744=CARTESIAN_POINT ( 'NONE',  ( -3.749999999999997780, -7.438900925035489387, 24.09561829374151287 ) ) ;
#68752=CARTESIAN_POINT ( 'NONE',  ( 2.651650429449539104, -4.848349570550432475, 14.31250000000000000 ) ) ;
#68831=CARTESIAN_POINT ( 'NONE',  ( 3.749999999999992006, -5.946699141100872943, 24.39062500000000000 ) ) ;
#68840=CARTESIAN_POINT ( 'NONE',  ( 3.724691934501232815, -5.885600066136343678, 17.88875670625848713 ) ) ;
#68856=CARTESIAN_POINT ( 'NONE',  ( 2.724691934501250135, -8.700186371490531201, 23.54874329374151642 ) ) ;
#68862=CARTESIAN_POINT ( 'NONE',  ( 2.750000000000008438, -8.639087296525996607, 22.04687500000000000 ) ) ;
#68943=CARTESIAN_POINT ( 'NONE',  ( -2.651650429449535551, -10.15165042944956753, 14.93750000000000000 ) ) ;
#68960=CARTESIAN_POINT ( 'NONE',  ( -2.775308065498752086, -8.577988221561495763, 19.01749329374151287 ) ) ;
#69071=CARTESIAN_POINT ( 'NONE',  ( -1.944543648263014957, -5.555456351737005249, 17.75000000000000355 ) ) ;
#69137=CARTESIAN_POINT ( 'NONE',  ( 2.320192649118979489E-14, -11.25000000000000000, 19.78125000000000000 ) ) ;
#69172=CARTESIAN_POINT ( 'NONE',  ( 1.901340078031349856, -5.512252781505337929, 16.56063170625848713 ) ) ;
#69182=CARTESIAN_POINT ( 'NONE',  ( -0.06109907496454585613, -4.750000000000000000, 17.65438170625849068 ) ) ;
#69189=CARTESIAN_POINT ( 'NONE',  ( -3.775308065498748977, -8.992201783934593351, 25.26749329374151642 ) ) ;
#69195=CARTESIAN_POINT ( 'NONE',  ( 2.320192649118979489E-14, -11.25000000000000000, 14.78125000000000178 ) ) ;
#69281=CARTESIAN_POINT ( 'NONE',  ( -0.06109907496455085213, -3.750000000000000888, 16.40438170625849068 ) ) ;
#69290=CARTESIAN_POINT ( 'NONE',  ( -3.749999999999988454, -9.053300858899127945, 26.26562500000000000 ) ) ;
#69308=CARTESIAN_POINT ( 'NONE',  ( 2.750000000000002665, -7.561099074964516831, 23.47061829374151642 ) ) ;
#69397=CARTESIAN_POINT ( 'NONE',  ( 2.651650429449539104, -4.848349570550432475, 14.31250000000000000 ) ) ;
#69410=CARTESIAN_POINT ( 'NONE',  ( 3.750000000000001776, -7.561099074964511502, 14.72061829374151465 ) ) ;
#69495=EDGE_LOOP ( 'NONE', ( #80643, #1084, #45841, #63295, #67237, #81499 ) ) ;
#69509=CARTESIAN_POINT ( 'NONE',  ( -1.409462824231155764E-14, -4.749999999999999112, 25.40625000000000000 ) ) ;
#69526=CARTESIAN_POINT ( 'NONE',  ( 3.750000000000000888, -7.499999999999978684, 25.71875000000000000 ) ) ;
#69577=CARTESIAN_POINT ( 'NONE',  ( 1.553300858899129722, -11.24999999999999112, 24.70312500000000000 ) ) ;
#69609=CARTESIAN_POINT ( 'NONE',  ( 1.901340078031349856, -5.512252781505337929, 17.81063170625849068 ) ) ;
#69619=CARTESIAN_POINT ( 'NONE',  ( 1.200186371490561621, -10.22469193450123193, 16.95125670625848713 ) ) ;
#69629=CARTESIAN_POINT ( 'NONE',  ( 1.492201783934598236, -11.27530806549875031, 24.95499329374151287 ) ) ;
#69633=CARTESIAN_POINT ( 'NONE',  ( 0.06109907496451268821, -3.749999999999999556, 23.15811829374151642 ) ) ;
#69719=CARTESIAN_POINT ( 'NONE',  ( 3.749999999999992006, -5.946699141100872943, 25.64062500000000000 ) ) ;
#69728=CARTESIAN_POINT ( 'NONE',  ( -0.06109907496455085213, -3.750000000000000888, 15.15438170625848890 ) ) ;
#69743=CARTESIAN_POINT ( 'NONE',  ( -1.901340078031369618, -5.512252781505359245, 21.75186829374151287 ) ) ;
#69852=CARTESIAN_POINT ( 'NONE',  ( -2.694853999681181556, -10.10844685921792241, 13.93936829374151465 ) ) ;
#69860=CARTESIAN_POINT ( 'NONE',  ( -1.944543648263014957, -5.555456351737005249, 15.25000000000000000 ) ) ;
#69912=UNCERTAINTY_MEASURE_WITH_UNIT (LENGTH_MEASURE( 1.000000000000000082E-05 ), #73083, 'distance_accuracy_value', 'NONE');
#69952=CARTESIAN_POINT ( 'NONE',  ( -1.944543648263014957, -5.555456351737005249, 25.25000000000000000 ) ) ;
#70052=CARTESIAN_POINT ( 'NONE',  ( -1.901340078031346525, -9.487747218494661183, 22.18563170625848713 ) ) ;
#70054=CARTESIAN_POINT ( 'NONE',  ( -1.980058552680825423, -4.310325471588868140, 13.99999999999999289 ) ) ;
#70065=CARTESIAN_POINT ( 'NONE',  ( -1.987747218494660295, -5.598659921968651254, 24.99813170625849423 ) ) ;
#70074=CARTESIAN_POINT ( 'NONE',  ( 3.750000000000009770, -9.053300858899081760, 18.29687500000000000 ) ) ;
#70079=CARTESIAN_POINT ( 'NONE',  ( 3.775308065498752086, -6.007798216065404873, 24.64249329374151642 ) ) ;
#70160=CARTESIAN_POINT ( 'NONE',  ( -2.608446859217889546, -10.19485399968121264, 19.68563170625849068 ) ) ;
#70172=CARTESIAN_POINT ( 'NONE',  ( -3.775308065498766297, -6.007798216065450170, 16.17000670625848713 ) ) ;
#70185=CARTESIAN_POINT ( 'NONE',  ( -0.06109907496451398579, -10.25000000000000178, 22.53311829374151642 ) ) ;
#70293=CARTESIAN_POINT ( 'NONE',  ( -3.749999999999997780, -7.438900925035489387, 14.09561829374151642 ) ) ;
#70298=CARTESIAN_POINT ( 'NONE',  ( -1.944543648262992530, -9.444543648263016067, 18.68750000000000000 ) ) ;
#70302=CARTESIAN_POINT ( 'NONE',  ( 1.139087296526029469, -10.24999999999999289, 15.95312499999999822 ) ) ;
#70406=CARTESIAN_POINT ( 'NONE',  ( 1.944543648263018731, -9.444543648262994751, 22.12500000000000000 ) ) ;
#70407=ORIENTED_EDGE ( 'NONE', *, *, #18440, .F. ) ;
#70471=CARTESIAN_POINT ( 'NONE',  ( 1.553300858899086867, -3.749999999999992006, 24.23437500000000355 ) ) ;
#70500=CARTESIAN_POINT ( 'NONE',  ( 0.06109907496454976272, -10.25000000000000000, 23.27938170625849068 ) ) ;
#70513=CARTESIAN_POINT ( 'NONE',  ( 1.077988221561464899, -4.724691934501233703, 22.73250670625849068 ) ) ;
#70523=CARTESIAN_POINT ( 'NONE',  ( -2.651650429449565305, -4.848349570550461785, 14.00000000000000000 ) ) ;
#70527=CARTESIAN_POINT ( 'NONE',  ( -3.749999999999988454, -9.053300858899127945, 17.51562500000000000 ) ) ;
#70529=DIRECTION ( 'NONE',  ( 0.7071067811865510144, -0.7071067811865441310, 0.000000000000000000 ) ) ;
#70607=CARTESIAN_POINT ( 'NONE',  ( 3.724691934501232815, -5.885600066136343678, 20.38875670625849068 ) ) ;
#70615=CARTESIAN_POINT ( 'NONE',  ( -3.775308065498766297, -6.007798216065450170, 21.17000670625848713 ) ) ;
#70630=CARTESIAN_POINT ( 'NONE',  ( 2.750000000000002665, -7.561099074964516831, 24.72061829374150932 ) ) ;
#70716=CARTESIAN_POINT ( 'NONE',  ( 3.750000000000000888, -7.499999999999978684, 16.96875000000000000 ) ) ;
#70726=CARTESIAN_POINT ( 'NONE',  ( -2.651650429449565305, -4.848349570550461785, 19.00000000000000000 ) ) ;
#70741=CARTESIAN_POINT ( 'NONE',  ( 3.775308065498752086, -6.007798216065404873, 14.64249329374151110 ) ) ;
#70745=CARTESIAN_POINT ( 'NONE',  ( -1.944543648263014957, -5.555456351737005249, 20.25000000000000000 ) ) ;
#70749=CARTESIAN_POINT ( 'NONE',  ( 1.944543648262996083, -5.555456351736983045, 14.31250000000000000 ) ) ;
#70796=AXIS2_PLACEMENT_3D ( 'NONE', #42630, #17709, #29995 ) ;
#70807=PRODUCT_DEFINITION_CONTEXT ( 'detailed design', #26811, 'design' ) ;
#70852=CARTESIAN_POINT ( 'NONE',  ( 1.799775606325937360E-14, -10.25000000000000000, 23.53125000000000000 ) ) ;
#70915=CARTESIAN_POINT ( 'NONE',  ( 2.651650429449569302, -10.15165042944953733, 23.37500000000000000 ) ) ;
#70944=CARTESIAN_POINT ( 'NONE',  ( 1.901340078031349856, -5.512252781505337929, 21.56063170625849068 ) ) ;
#70947=CARTESIAN_POINT ( 'NONE',  ( 2.410688644434096695, -4.750108984206948826, 14.00000000000000533 ) ) ;
#70955=CARTESIAN_POINT ( 'NONE',  ( 2.775308065498768517, -8.577988221561467341, 25.54500670625849779 ) ) ;
#70963=CARTESIAN_POINT ( 'NONE',  ( -2.651650429449535551, -10.15165042944956753, 16.18750000000000000 ) ) ;
#70970=CARTESIAN_POINT ( 'NONE',  ( 1.553300858899087311, -3.749999999999992006, 15.48437500000000178 ) ) ;
#71006=CARTESIAN_POINT ( 'NONE',  ( -1.929879867024197893E-14, -3.750000000000000000, 21.65625000000000355 ) ) ;
#71045=CARTESIAN_POINT ( 'NONE',  ( -3.749999999999996447, -7.561099074964554134, 21.09188170625849068 ) ) ;
#71052=CARTESIAN_POINT ( 'NONE',  ( -3.724691934501229262, -9.114399933863657211, 22.26375670625849068 ) ) ;
#71068=CARTESIAN_POINT ( 'NONE',  ( 1.901340078031373171, -9.487747218494639867, 24.87686829374151642 ) ) ;
#71144=CARTESIAN_POINT ( 'NONE',  ( -1.929879867024197893E-14, -3.750000000000000000, 17.90625000000000000 ) ) ;
#71154=CARTESIAN_POINT ( 'NONE',  ( -1.553300858899125059, -3.750000000000009326, 19.07812500000000000 ) ) ;
#71168=CARTESIAN_POINT ( 'NONE',  ( 2.775308065498755195, -6.422011778438505125, 24.64249329374151642 ) ) ;
#71172=CARTESIAN_POINT ( 'NONE',  ( 1.139087296525997273, -4.749999999999992895, 25.48437500000000000 ) ) ;
#71178=CARTESIAN_POINT ( 'NONE',  ( -1.944543648263015179, -5.555456351737005249, 14.00000000000000000 ) ) ;
#71266=CARTESIAN_POINT ( 'NONE',  ( -2.749999999999991562, -8.639087296526025028, 23.76562499999999645 ) ) ;
#71343=CARTESIAN_POINT ( 'NONE',  ( 3.750000000000009770, -9.053300858899081760, 25.79687500000000355 ) ) ;
#71373=CARTESIAN_POINT ( 'NONE',  ( -2.724691934501232371, -8.700186371490559623, 21.01375670625849068 ) ) ;
#71375=CARTESIAN_POINT ( 'NONE',  ( 3.163032119165662515, -5.792891488981608994, 14.00000000000015099 ) ) ;
#71385=CARTESIAN_POINT ( 'NONE',  ( -1.901340078031346525, -9.487747218494661183, 24.68563170625849068 ) ) ;
#71394=CARTESIAN_POINT ( 'NONE',  ( 1.553300858899087311, -3.749999999999992006, 14.23437500000000355 ) ) ;
#71399=CARTESIAN_POINT ( 'NONE',  ( -1.553300858899081538, -11.25000000000000711, 16.10937500000000355 ) ) ;
#71438=CARTESIAN_POINT ( 'NONE',  ( -2.651650429449535551, -10.15165042944956753, 22.43750000000000000 ) ) ;
#71478=CARTESIAN_POINT ( 'NONE',  ( -2.694853999681210865, -4.891553140782108677, 18.74813170625849068 ) ) ;
#71488=CARTESIAN_POINT ( 'NONE',  ( 1.492201783934554493, -3.724691934501233703, 20.23250670625849423 ) ) ;
#71503=CARTESIAN_POINT ( 'NONE',  ( 3.775308065498752086, -6.007798216065404873, 15.89249329374151820 ) ) ;
#71582=CARTESIAN_POINT ( 'NONE',  ( 3.750000000000009770, -9.053300858899081760, 18.29687500000000000 ) ) ;
#71591=CARTESIAN_POINT ( 'NONE',  ( -3.749999999999988454, -9.053300858899127945, 20.01562500000000355 ) ) ;
#71606=CARTESIAN_POINT ( 'NONE',  ( -3.775308065498748977, -8.992201783934593351, 17.76749329374151287 ) ) ;
#71612=CARTESIAN_POINT ( 'NONE',  ( 2.724691934501250135, -8.700186371490531201, 13.54874329374151465 ) ) ;
#71617=CARTESIAN_POINT ( 'NONE',  ( -2.750000000000006217, -6.360912703474006946, 17.67187500000000355 ) ) ;
#71658=ORIENTED_EDGE ( 'NONE', *, *, #81056, .F. ) ;
#71714=CARTESIAN_POINT ( 'NONE',  ( 0.06109907496451789238, -4.749999999999998224, 15.65811829374151287 ) ) ;
#71823=CARTESIAN_POINT ( 'NONE',  ( -1.987747218494660295, -5.598659921968651254, 23.74813170625849068 ) ) ;
#71824=EDGE_LOOP ( 'NONE', ( #71658, #42396, #72412 ) ) ;
#71834=CARTESIAN_POINT ( 'NONE',  ( 0.06109907496454976272, -10.25000000000000000, 24.52938170625849423 ) ) ;
#71844=CARTESIAN_POINT ( 'NONE',  ( 3.749999999999992006, -5.946699141100872943, 15.64062500000000178 ) ) ;
#71848=CARTESIAN_POINT ( 'NONE',  ( -2.651650429449565305, -4.848349570550461785, 19.00000000000000000 ) ) ;
#71887=CARTESIAN_POINT ( 'NONE',  ( 3.750000000000000888, -7.499999999999978684, 20.71875000000000000 ) ) ;
#71927=CARTESIAN_POINT ( 'NONE',  ( -2.694853999681210865, -4.891553140782108677, 19.99813170625848713 ) ) ;
#71938=CARTESIAN_POINT ( 'NONE',  ( -2.694853999681210865, -4.891553140782108677, 18.74813170625849068 ) ) ;
#71952=CARTESIAN_POINT ( 'NONE',  ( -2.724691934501246582, -6.299813628509474128, 25.42374329374151998 ) ) ;
#72029=CARTESIAN_POINT ( 'NONE',  ( -3.749999999999988454, -9.053300858899127945, 15.01562500000000178 ) ) ;
#72040=CARTESIAN_POINT ( 'NONE',  ( -1.553300858899081538, -11.25000000000000711, 17.35937500000000000 ) ) ;
#72055=CARTESIAN_POINT ( 'NONE',  ( -1.492201783934593573, -3.724691934501250135, 18.07999329374151287 ) ) ;
#72061=CARTESIAN_POINT ( 'NONE',  ( -2.749999999999991562, -8.639087296526025028, 25.01562500000000000 ) ) ;
#72066=CARTESIAN_POINT ( 'NONE',  ( 2.749999999999995115, -6.360912703473971419, 18.14062500000000355 ) ) ;
#72159=( GEOMETRIC_REPRESENTATION_CONTEXT ( 3 ) GLOBAL_UNCERTAINTY_ASSIGNED_CONTEXT ( ( #28093 ) ) GLOBAL_UNIT_ASSIGNED_CONTEXT ( ( #47359, #74399, #27543 ) ) REPRESENTATION_CONTEXT ( 'NONE', 'WORKASPACE' ) );
#72160=CARTESIAN_POINT ( 'NONE',  ( 0.06109907496451789238, -4.749999999999998224, 16.90811829374151287 ) ) ;
#72269=CARTESIAN_POINT ( 'NONE',  ( -1.077988221561460236, -10.27530806549876452, 27.10750670625849423 ) ) ;
#72271=CARTESIAN_POINT ( 'NONE',  ( 2.836344605459119261, -5.235657397115412337, 14.00000000000008882 ) ) ;
#72278=CARTESIAN_POINT ( 'NONE',  ( 1.944543648262996083, -5.555456351736983045, 16.81250000000000000 ) ) ;
#72286=CARTESIAN_POINT ( 'NONE',  ( 3.750000000000000888, -7.499999999999978684, 21.96875000000000355 ) ) ;
#72316=AXIS2_PLACEMENT_3D ( 'NONE', #52266, #18049, #23894 ) ;
#72330=CARTESIAN_POINT ( 'NONE',  ( -2.651650429449565305, -4.848349570550461785, 21.50000000000000000 ) ) ;
#72337=CARTESIAN_POINT ( 'NONE',  ( -1.553300858899081760, -11.25000000000000888, 17.35937499999999645 ) ) ;
#72369=CARTESIAN_POINT ( 'NONE',  ( -3.724691934501229262, -9.114399933863657211, 26.01375670625848713 ) ) ;
#72377=CARTESIAN_POINT ( 'NONE',  ( 2.608446859217893099, -4.805146000318787358, 20.31063170625848713 ) ) ;
#72391=CARTESIAN_POINT ( 'NONE',  ( 1.614399933863618797, -3.775308065498751198, 14.48624329374151465 ) ) ;
#72412=ORIENTED_EDGE ( 'NONE', *, *, #28885, .F. ) ;
#72476=CARTESIAN_POINT ( 'NONE',  ( -1.553300858899081538, -11.25000000000000711, 17.35937500000000000 ) ) ;
#72486=CARTESIAN_POINT ( 'NONE',  ( -1.929879867024197893E-14, -3.750000000000000000, 15.40625000000000000 ) ) ;
#72504=CARTESIAN_POINT ( 'NONE',  ( 1.077988221561497539, -10.27530806549875386, 13.70499329374151287 ) ) ;
#72510=CARTESIAN_POINT ( 'NONE',  ( 2.750000000000001776, -7.499999999999984013, 20.71875000000000000 ) ) ;
#72607=CARTESIAN_POINT ( 'NONE',  ( 1.901340078031373171, -9.487747218494639867, 16.12686829374151287 ) ) ;
#72632=PRESENTATION_STYLE_ASSIGNMENT (( #79403 ) ) ;
#72714=CARTESIAN_POINT ( 'NONE',  ( -1.409462824231155764E-14, -4.749999999999999112, 15.40625000000000000 ) ) ;
#72722=CARTESIAN_POINT ( 'NONE',  ( -1.200186371490556958, -4.775308065498765409, 26.32625670625849068 ) ) ;
#72730=CARTESIAN_POINT ( 'NONE',  ( 3.749999999999992006, -5.946699141100872943, 19.39062500000000711 ) ) ;
#72778=CARTESIAN_POINT ( 'NONE',  ( 3.750000000000009770, -9.053300858899081760, 15.79687500000000178 ) ) ;
#72795=CARTESIAN_POINT ( 'NONE',  ( 2.952004793765244717, -6.965521097154411478, 14.00000000000000178 ) ) ;
#72812=CARTESIAN_POINT ( 'NONE',  ( 3.775308065498768517, -8.992201783934554271, 25.54500670625849779 ) ) ;
#72820=CARTESIAN_POINT ( 'NONE',  ( 2.750000000000001332, -7.438900925035452083, 15.46688170625848713 ) ) ;
#72836=CARTESIAN_POINT ( 'NONE',  ( 2.608446859217924629, -10.19485399968118422, 19.87686829374151287 ) ) ;
#72927=CARTESIAN_POINT ( 'NONE',  ( -2.651650429449565305, -4.848349570550461785, 22.75000000000000000 ) ) ;
#72937=CARTESIAN_POINT ( 'NONE',  ( -1.553300858899125059, -3.750000000000009326, 24.07812500000000355 ) ) ;
#72956=CARTESIAN_POINT ( 'NONE',  ( -1.139087296526025916, -4.750000000000006217, 22.82812500000000355 ) ) ;
#72962=CARTESIAN_POINT ( 'NONE',  ( 1.139087296526029469, -10.24999999999999289, 18.45312499999999645 ) ) ;
#73037=SHAPE_DEFINITION_REPRESENTATION ( #41210, #11000 ) ;
#73058=CARTESIAN_POINT ( 'NONE',  ( -0.06109907496451398579, -10.25000000000000178, 17.53311829374151287 ) ) ;
#73083=( LENGTH_UNIT ( ) NAMED_UNIT ( * ) SI_UNIT ( .MILLI., .METRE. ) );
#73171=CARTESIAN_POINT ( 'NONE',  ( -2.749999999999997780, -7.561099074964547917, 27.34188170625848713 ) ) ;
#73181=CARTESIAN_POINT ( 'NONE',  ( -1.944543648262992530, -9.444543648263016067, 17.43750000000000000 ) ) ;
#73189=CARTESIAN_POINT ( 'NONE',  ( -3.750000000000008438, -5.946699141100917352, 18.92187500000000355 ) ) ;
#73250=CARTESIAN_POINT ( 'NONE',  ( -2.102533092329708531, -5.360057338231124291, 13.56786352175840626 ) ) ;
#73267=CARTESIAN_POINT ( 'NONE',  ( -1.492201783934549164, -11.27530806549876807, 25.85750670625849068 ) ) ;
#73280=CARTESIAN_POINT ( 'NONE',  ( -1.077988221561460236, -10.27530806549876452, 15.85750670625849068 ) ) ;
#73295=CARTESIAN_POINT ( 'NONE',  ( 3.775308065498752086, -6.007798216065404873, 20.89249329374151642 ) ) ;
#73376=CARTESIAN_POINT ( 'NONE',  ( 2.320192649118979489E-14, -11.25000000000000000, 19.78125000000000000 ) ) ;
#73387=CARTESIAN_POINT ( 'NONE',  ( 2.320192649118979489E-14, -11.25000000000000000, 24.78125000000000000 ) ) ;
#73405=CARTESIAN_POINT ( 'NONE',  ( 2.750000000000002665, -7.561099074964516831, 14.72061829374151465 ) ) ;
#73414=CARTESIAN_POINT ( 'NONE',  ( 1.944543648262996083, -5.555456351736983045, 18.06250000000000355 ) ) ;
#73514=CARTESIAN_POINT ( 'NONE',  ( 2.724691934501250135, -8.700186371490531201, 13.54874329374151465 ) ) ;
#73515=VERTEX_POINT ( 'NONE', #6604 ) ;
#73631=CARTESIAN_POINT ( 'NONE',  ( -2.750000000000007105, -6.360912703474006946, 16.42187500000000000 ) ) ;
#73639=CARTESIAN_POINT ( 'NONE',  ( 2.750000000000001776, -7.499999999999984013, 15.71875000000000000 ) ) ;
#73648=CARTESIAN_POINT ( 'NONE',  ( 1.553300858899129944, -11.24999999999998934, 19.70312500000000355 ) ) ;
#73688=CARTESIAN_POINT ( 'NONE',  ( -1.553300858899081538, -11.25000000000000711, 24.85937500000001421 ) ) ;
#73694=CARTESIAN_POINT ( 'NONE',  ( -2.651650429449565305, -4.848349570550461785, 17.75000000000000355 ) ) ;
#73727=CARTESIAN_POINT ( 'NONE',  ( 2.694853999681214862, -10.10844685921789043, 25.62313170625849068 ) ) ;
#73740=CARTESIAN_POINT ( 'NONE',  ( -1.492201783934549164, -11.27530806549876807, 24.60750670625849779 ) ) ;
#73748=CARTESIAN_POINT ( 'NONE',  ( 3.775308065498752086, -6.007798216065404873, 17.14249329374151287 ) ) ;
#73756=CARTESIAN_POINT ( 'NONE',  ( -3.749999999999997780, -7.438900925035489387, 19.09561829374150932 ) ) ;
#73833=CARTESIAN_POINT ( 'NONE',  ( 3.749999999999992006, -5.946699141100872943, 20.64062500000000000 ) ) ;
#73841=CARTESIAN_POINT ( 'NONE',  ( 1.553300858899129944, -11.24999999999998934, 22.20312500000000000 ) ) ;
#73857=CARTESIAN_POINT ( 'NONE',  ( -1.987747218494638313, -9.401340078031370950, 17.68936829374151287 ) ) ;
#73863=CARTESIAN_POINT ( 'NONE',  ( -1.944543648263014957, -5.555456351737005249, 22.75000000000000000 ) ) ;
#73957=CARTESIAN_POINT ( 'NONE',  ( 0.06109907496451789238, -4.749999999999998224, 20.65811829374151287 ) ) ;
#74065=CARTESIAN_POINT ( 'NONE',  ( 1.077988221561464899, -4.724691934501233703, 25.23250670625849068 ) ) ;
#74074=CARTESIAN_POINT ( 'NONE',  ( 2.750000000000008438, -8.639087296525996607, 15.79687500000000178 ) ) ;
#74081=CARTESIAN_POINT ( 'NONE',  ( -3.750000000000008438, -5.946699141100917352, 21.42187500000000000 ) ) ;
#74125=CARTESIAN_POINT ( 'NONE',  ( -2.651650429449535551, -10.15165042944956753, 21.18750000000000000 ) ) ;
#74157=CARTESIAN_POINT ( 'NONE',  ( -3.775308065498766297, -6.007798216065450170, 23.67000670625849779 ) ) ;
#74169=CARTESIAN_POINT ( 'NONE',  ( 3.724691934501232815, -5.885600066136343678, 26.63875670625848713 ) ) ;
#74176=CARTESIAN_POINT ( 'NONE',  ( -3.749999999999997780, -7.438900925035489387, 16.59561829374151287 ) ) ;
#74182=CARTESIAN_POINT ( 'NONE',  ( 1.492201783934598236, -11.27530806549875031, 17.45499329374151642 ) ) ;
#74184=FACE_OUTER_BOUND ( 'NONE', #57786, .T. ) ;
#74268=CARTESIAN_POINT ( 'NONE',  ( 1.553300858899129944, -11.24999999999998934, 23.45312500000000000 ) ) ;
#74277=CARTESIAN_POINT ( 'NONE',  ( -1.929879867024197893E-14, -3.750000000000000000, 20.40625000000000000 ) ) ;
#74293=CARTESIAN_POINT ( 'NONE',  ( -0.06109907496451398579, -10.25000000000000178, 16.28311829374151287 ) ) ;
#74299=CARTESIAN_POINT ( 'NONE',  ( -1.409462824231155764E-14, -4.749999999999999112, 24.15625000000000000 ) ) ;
#74394=CARTESIAN_POINT ( 'NONE',  ( -1.200186371490524317, -10.22469193450124791, 18.86124329374151287 ) ) ;
#74399=( NAMED_UNIT ( * ) PLANE_ANGLE_UNIT ( ) SI_UNIT ( $, .RADIAN. ) );
#74498=CARTESIAN_POINT ( 'NONE',  ( 1.799775606325937360E-14, -10.25000000000000000, 19.78125000000000000 ) ) ;
#74509=CARTESIAN_POINT ( 'NONE',  ( 1.799775606325937360E-14, -10.25000000000000000, 18.53125000000000000 ) ) ;
#74572=CARTESIAN_POINT ( 'NONE',  ( -1.553300858899081760, -11.25000000000000888, 21.10937500000000000 ) ) ;
#74602=CARTESIAN_POINT ( 'NONE',  ( 1.077988221561464899, -4.724691934501233703, 18.98250670625849068 ) ) ;
#74614=CARTESIAN_POINT ( 'NONE',  ( 1.077988221561464899, -4.724691934501233703, 18.98250670625849068 ) ) ;
#74623=CARTESIAN_POINT ( 'NONE',  ( 1.614399933863618797, -3.775308065498751198, 19.48624329374152353 ) ) ;
#74629=CARTESIAN_POINT ( 'NONE',  ( -3.749999999999997780, -7.438900925035489387, 16.59561829374151287 ) ) ;
#74701=STYLED_ITEM ( 'NONE', ( #518 ), #9 ) ;
#74719=CARTESIAN_POINT ( 'NONE',  ( -3.750000000000008438, -5.946699141100917352, 25.17187500000000000 ) ) ;
#74727=CARTESIAN_POINT ( 'NONE',  ( 3.750000000000000888, -7.499999999999978684, 20.71875000000000000 ) ) ;
#74745=CARTESIAN_POINT ( 'NONE',  ( -1.200186371490524317, -10.22469193450124791, 16.36124329374151642 ) ) ;
#74751=CARTESIAN_POINT ( 'NONE',  ( 2.749999999999995115, -6.360912703473971419, 24.39062500000000000 ) ) ;
#74849=CARTESIAN_POINT ( 'NONE',  ( 1.200186371490529202, -4.775308065498752974, 21.98624329374151642 ) ) ;
#74955=CARTESIAN_POINT ( 'NONE',  ( 2.750000000000001776, -7.499999999999984013, 18.21875000000000000 ) ) ;
#74964=CARTESIAN_POINT ( 'NONE',  ( 1.944543648262996083, -5.555456351736983045, 18.06250000000000355 ) ) ;
#75020=CARTESIAN_POINT ( 'NONE',  ( -3.749999999999997335, -7.500000000000021316, 20.09375000000000000 ) ) ;
#75051=CARTESIAN_POINT ( 'NONE',  ( 1.901340078031349856, -5.512252781505337929, 19.06063170625849068 ) ) ;
#75064=CARTESIAN_POINT ( 'NONE',  ( -1.200186371490556958, -4.775308065498765409, 17.57625670625849068 ) ) ;
#75071=CARTESIAN_POINT ( 'NONE',  ( -2.608446859217920633, -4.805146000318815780, 23.00186829374151287 ) ) ;
#75075=CARTESIAN_POINT ( 'NONE',  ( -1.614399933863613468, -11.22469193450124969, 25.11124329374151642 ) ) ;
#75160=CARTESIAN_POINT ( 'NONE',  ( 1.553300858899129944, -11.24999999999998934, 25.95312500000000000 ) ) ;
#75170=CARTESIAN_POINT ( 'NONE',  ( 2.651650429449539104, -4.848349570550432475, 25.56250000000000355 ) ) ;
#75185=CARTESIAN_POINT ( 'NONE',  ( 1.200186371490529202, -4.775308065498752974, 16.98624329374151287 ) ) ;
#75192=CARTESIAN_POINT ( 'NONE',  ( -1.139087296525992388, -10.25000000000000711, 23.60937500000000711 ) ) ;
#75285=CARTESIAN_POINT ( 'NONE',  ( -1.987747218494638313, -9.401340078031370950, 18.93936829374151287 ) ) ;
#75341=CARTESIAN_POINT ( 'NONE',  ( -3.749999999999997335, -7.500000000000021316, 25.09374999999999645 ) ) ;
#75387=CARTESIAN_POINT ( 'NONE',  ( 1.799775606325937360E-14, -10.25000000000000000, 21.03125000000000000 ) ) ;
#75396=CARTESIAN_POINT ( 'NONE',  ( 1.139087296526029469, -10.24999999999999467, 20.95312500000000000 ) ) ;
#75405=CARTESIAN_POINT ( 'NONE',  ( -1.929879867024197893E-14, -3.750000000000000000, 25.40625000000000000 ) ) ;
#75452=CARTESIAN_POINT ( 'NONE',  ( 3.750000000000009770, -9.053300858899081760, 20.79687500000000000 ) ) ;
#75478=CARTESIAN_POINT ( 'NONE',  ( 2.724691934501235036, -6.299813628509441266, 17.88875670625848713 ) ) ;
#75489=CARTESIAN_POINT ( 'NONE',  ( -0.06109907496454585613, -4.750000000000000000, 16.40438170625849068 ) ) ;
#75498=CARTESIAN_POINT ( 'NONE',  ( 3.775308065498752086, -6.007798216065404873, 20.89249329374151642 ) ) ;
#75504=CARTESIAN_POINT ( 'NONE',  ( -1.492201783934593573, -3.724691934501250135, 24.32999329374151642 ) ) ;
#75582=CARTESIAN_POINT ( 'NONE',  ( 1.492201783934554493, -3.724691934501233703, 15.23250670625848713 ) ) ;
#75590=CARTESIAN_POINT ( 'NONE',  ( 0.06109907496455496689, -11.24999999999999822, 18.27938170625849068 ) ) ;
#75605=CARTESIAN_POINT ( 'NONE',  ( 1.987747218494642309, -5.598659921968629050, 19.56436829374151287 ) ) ;
#75612=CARTESIAN_POINT ( 'NONE',  ( -1.139087296525992388, -10.25000000000000711, 26.10937500000000355 ) ) ;
#75712=CARTESIAN_POINT ( 'NONE',  ( -2.724691934501246582, -6.299813628509474128, 20.42374329374152353 ) ) ;
#75822=CARTESIAN_POINT ( 'NONE',  ( -1.139087296526025916, -4.750000000000006217, 21.57812500000000355 ) ) ;
#75832=CARTESIAN_POINT ( 'NONE',  ( 2.750000000000008438, -8.639087296525996607, 20.79687500000000000 ) ) ;
#75841=CARTESIAN_POINT ( 'NONE',  ( 2.320192649118979489E-14, -11.25000000000000000, 26.03125000000000000 ) ) ;
#75894=CARTESIAN_POINT ( 'NONE',  ( -1.929879867024197893E-14, -3.750000000000000000, 20.40625000000000000 ) ) ;
#75927=CARTESIAN_POINT ( 'NONE',  ( -2.749999999999997780, -7.561099074964547917, 16.09188170625848713 ) ) ;
#75938=CARTESIAN_POINT ( 'NONE',  ( 1.987747218494664292, -9.401340078031346081, 16.87313170625849068 ) ) ;
#75946=CARTESIAN_POINT ( 'NONE',  ( 0.06109907496451268821, -3.749999999999999556, 23.15811829374151642 ) ) ;
#75954=CARTESIAN_POINT ( 'NONE',  ( -1.929879867024197893E-14, -3.750000000000000000, 14.15625000000000000 ) ) ;
#76029=CARTESIAN_POINT ( 'NONE',  ( -2.694853999681210865, -4.891553140782108677, 14.99813170625848713 ) ) ;
#76038=CARTESIAN_POINT ( 'NONE',  ( -2.651650429449535551, -10.15165042944956753, 26.18750000000000355 ) ) ;
#76054=CARTESIAN_POINT ( 'NONE',  ( 1.987747218494642309, -5.598659921968629050, 22.06436829374151287 ) ) ;
#76156=CARTESIAN_POINT ( 'NONE',  ( -3.724691934501248802, -5.885600066136383646, 14.17374329374151287 ) ) ;
#76261=CARTESIAN_POINT ( 'NONE',  ( -1.944543648263014957, -5.555456351737005249, 24.00000000000000000 ) ) ;
#76279=CARTESIAN_POINT ( 'NONE',  ( 2.651650429449539104, -4.848349570550432475, 25.56250000000000355 ) ) ;
#76333=CARTESIAN_POINT ( 'NONE',  ( -3.749999999999988454, -9.053300858899127945, 26.26562500000000000 ) ) ;
#76364=CARTESIAN_POINT ( 'NONE',  ( -1.987747218494660295, -5.598659921968651254, 19.99813170625848713 ) ) ;
#76377=CARTESIAN_POINT ( 'NONE',  ( -1.901340078031346525, -9.487747218494661183, 20.93563170625849068 ) ) ;
#76387=CARTESIAN_POINT ( 'NONE',  ( -0.06109907496450878162, -11.25000000000000000, 25.03311829374151287 ) ) ;
#76394=CARTESIAN_POINT ( 'NONE',  ( -0.06109907496450878162, -11.25000000000000000, 23.78311829374151998 ) ) ;
#76482=CARTESIAN_POINT ( 'NONE',  ( 1.492201783934554493, -3.724691934501233703, 17.73250670625848713 ) ) ;
#76491=CARTESIAN_POINT ( 'NONE',  ( -1.492201783934549164, -11.27530806549876807, 17.10750670625848713 ) ) ;
#76505=CARTESIAN_POINT ( 'NONE',  ( -2.775308065498752086, -8.577988221561495763, 19.01749329374151287 ) ) ;
#76610=CARTESIAN_POINT ( 'NONE',  ( 2.724691934501250135, -8.700186371490531201, 24.79874329374151998 ) ) ;
#76717=CARTESIAN_POINT ( 'NONE',  ( -1.139087296525992166, -10.25000000000000533, 22.35937500000000711 ) ) ;
#76821=CARTESIAN_POINT ( 'NONE',  ( 1.077988221561464899, -4.724691934501233703, 21.48250670625849068 ) ) ;
#76825=VERTEX_POINT ( 'NONE', #53078 ) ;
#76834=CARTESIAN_POINT ( 'NONE',  ( 0.06109907496454976272, -10.25000000000000000, 22.02938170625849068 ) ) ;
#76842=CARTESIAN_POINT ( 'NONE',  ( -2.608446859217920633, -4.805146000318815780, 20.50186829374151287 ) ) ;
#76847=CARTESIAN_POINT ( 'NONE',  ( -3.749999999999997780, -7.438900925035489387, 24.09561829374151287 ) ) ;
#76924=CARTESIAN_POINT ( 'NONE',  ( -1.614399933863656544, -3.775308065498769405, 21.32625670625849423 ) ) ;
#76934=CARTESIAN_POINT ( 'NONE',  ( 2.694853999681214862, -10.10844685921789043, 16.87313170625849068 ) ) ;
#76948=CARTESIAN_POINT ( 'NONE',  ( -1.987747218494638313, -9.401340078031370950, 20.18936829374151287 ) ) ;
#77031=CARTESIAN_POINT ( 'NONE',  ( -1.553300858899125059, -3.750000000000009326, 14.07812500000000178 ) ) ;
#77056=CARTESIAN_POINT ( 'NONE',  ( 3.750000000000001776, -7.561099074964511502, 13.47061829374151465 ) ) ;
#77157=CARTESIAN_POINT ( 'NONE',  ( -1.139087296525992166, -10.25000000000000533, 23.60937500000000711 ) ) ;
#77220=CARTESIAN_POINT ( 'NONE',  ( -1.553300858899081760, -11.25000000000000888, 24.85937500000000711 ) ) ;
#77252=CARTESIAN_POINT ( 'NONE',  ( -1.077988221561460236, -10.27530806549876452, 22.10750670625849068 ) ) ;
#77254=CARTESIAN_POINT ( 'NONE',  ( -0.5647128961976267680, -3.802940288257858015, 13.99999999999966604 ) ) ;
#77265=CARTESIAN_POINT ( 'NONE',  ( 2.724691934501235036, -6.299813628509441266, 21.63875670625848713 ) ) ;
#77272=CARTESIAN_POINT ( 'NONE',  ( -3.749999999999997335, -7.500000000000021316, 18.84375000000000000 ) ) ;
#77278=CARTESIAN_POINT ( 'NONE',  ( -3.749999999999988454, -9.053300858899127945, 15.01562500000000178 ) ) ;
#77362=CARTESIAN_POINT ( 'NONE',  ( 2.694853999681214862, -10.10844685921789043, 19.37313170625848713 ) ) ;
#77370=CARTESIAN_POINT ( 'NONE',  ( 1.614399933863660985, -11.22469193450123193, 21.95125670625849068 ) ) ;
#77384=CARTESIAN_POINT ( 'NONE',  ( -1.200186371490524317, -10.22469193450124791, 25.11124329374151642 ) ) ;
#77468=CARTESIAN_POINT ( 'NONE',  ( -1.553300858899081538, -11.25000000000000711, 16.10937500000000355 ) ) ;
#77477=CARTESIAN_POINT ( 'NONE',  ( -3.749999999999997335, -7.500000000000021316, 18.84375000000000000 ) ) ;
#77489=CARTESIAN_POINT ( 'NONE',  ( 1.614399933863618797, -3.775308065498751198, 13.23624329374151465 ) ) ;
#77494=CARTESIAN_POINT ( 'NONE',  ( 1.944543648263018731, -9.444543648262994751, 19.62500000000000000 ) ) ;
#77498=CARTESIAN_POINT ( 'NONE',  ( -1.139087296526025250, -4.750000000000006217, 14.07812500000000178 ) ) ;
#77600=CARTESIAN_POINT ( 'NONE',  ( 2.750000000000001776, -7.499999999999984013, 21.96875000000000355 ) ) ;
#77661=CARTESIAN_POINT ( 'NONE',  ( -2.651650429449535551, -10.15165042944956753, 26.18750000000000355 ) ) ;
#77690=DIRECTION ( 'NONE',  ( 0.7071067811865510144, -0.7071067811865441310, 0.000000000000000000 ) ) ;
#77694=CARTESIAN_POINT ( 'NONE',  ( -0.06109907496454585613, -4.750000000000000000, 22.65438170625849068 ) ) ;
#77697=CARTESIAN_POINT ( 'NONE',  ( 3.105451396330338287, -7.707150910725261816, 14.00000000000000000 ) ) ;
#77706=CARTESIAN_POINT ( 'NONE',  ( -1.200186371490556958, -4.775308065498765409, 23.82625670625849068 ) ) ;
#77715=CARTESIAN_POINT ( 'NONE',  ( 2.651650429449539104, -4.848349570550432475, 15.56250000000000000 ) ) ;
#77719=CARTESIAN_POINT ( 'NONE',  ( -1.553300858899125059, -3.750000000000009326, 16.57812500000000000 ) ) ;
#77759=CARTESIAN_POINT ( 'NONE',  ( 2.320192649118979489E-14, -11.25000000000000000, 19.78125000000000000 ) ) ;
#77800=CARTESIAN_POINT ( 'NONE',  ( -1.492201783934549164, -11.27530806549876807, 18.35750670625849068 ) ) ;
#77807=CARTESIAN_POINT ( 'NONE',  ( 3.775308065498768517, -8.992201783934554271, 21.79500670625849068 ) ) ;
#77821=CARTESIAN_POINT ( 'NONE',  ( -3.749999999999997780, -7.438900925035489387, 14.09561829374151642 ) ) ;
#77904=CARTESIAN_POINT ( 'NONE',  ( 2.651650429449569302, -10.15165042944953733, 17.12500000000000000 ) ) ;
#77914=CARTESIAN_POINT ( 'NONE',  ( -2.651650429449565305, -4.848349570550461785, 17.75000000000000355 ) ) ;
#77929=CARTESIAN_POINT ( 'NONE',  ( -2.694853999681181556, -10.10844685921792241, 15.18936829374151465 ) ) ;
#77934=CARTESIAN_POINT ( 'NONE',  ( 1.944543648262996083, -5.555456351736983045, 24.31250000000000000 ) ) ;
#78036=CARTESIAN_POINT ( 'NONE',  ( -1.944543648263014957, -5.555456351737005249, 22.75000000000000000 ) ) ;
#78140=CARTESIAN_POINT ( 'NONE',  ( -1.200186371490556958, -4.775308065498765409, 25.07625670625849423 ) ) ;
#78143=CARTESIAN_POINT ( 'NONE',  ( 3.220692400827285695, -8.036656286327577448, 14.00000000000003908 ) ) ;
#78151=CARTESIAN_POINT ( 'NONE',  ( 0.06109907496454976272, -10.25000000000000000, 23.27938170625849068 ) ) ;
#78160=CARTESIAN_POINT ( 'NONE',  ( 2.651650429449569302, -10.15165042944953733, 15.87500000000000000 ) ) ;
#78165=CARTESIAN_POINT ( 'NONE',  ( -1.929879867024197893E-14, -3.750000000000000000, 17.90625000000000000 ) ) ;
#78168=DIRECTION ( 'NONE',  ( -0.7057856980126718804, -0.7057856980126787638, -0.06109907496453170772 ) ) ;
#78203=CARTESIAN_POINT ( 'NONE',  ( 3.750000000000009770, -9.053300858899081760, 23.29687500000000000 ) ) ;
#78239=CARTESIAN_POINT ( 'NONE',  ( -1.492201783934549164, -11.27530806549876807, 20.85750670625849068 ) ) ;
#78248=CARTESIAN_POINT ( 'NONE',  ( -3.775308065498766297, -6.007798216065450170, 22.42000670625849068 ) ) ;
#78262=CARTESIAN_POINT ( 'NONE',  ( -2.608446859217920633, -4.805146000318815780, 15.50186829374151287 ) ) ;
#78340=CARTESIAN_POINT ( 'NONE',  ( -1.553300858899125059, -3.750000000000009326, 17.82812500000000000 ) ) ;
#78351=CARTESIAN_POINT ( 'NONE',  ( -1.553300858899081538, -11.25000000000000711, 19.85937500000000355 ) ) ;
#78366=CARTESIAN_POINT ( 'NONE',  ( 2.694853999681185108, -4.891553140782077591, 17.06436829374151287 ) ) ;
#78367=ORIENTED_EDGE ( 'NONE', *, *, #81056, .T. ) ;
#78371=CARTESIAN_POINT ( 'NONE',  ( 2.775308065498755195, -6.422011778438505125, 13.39249329374151642 ) ) ;
#78376=CARTESIAN_POINT ( 'NONE',  ( 2.750000000000001776, -7.499999999999984013, 18.21875000000000000 ) ) ;
#78472=CARTESIAN_POINT ( 'NONE',  ( 1.077988221561497539, -10.27530806549875386, 14.95499329374151642 ) ) ;
#78581=CARTESIAN_POINT ( 'NONE',  ( 2.750000000000001332, -7.438900925035452083, 21.71688170625848713 ) ) ;
#78584=CARTESIAN_POINT ( 'NONE',  ( 1.732862688310258026, -4.223057123557754977, 14.00000000000000533 ) ) ;
#78592=CARTESIAN_POINT ( 'NONE',  ( -1.077988221561460236, -10.27530806549876452, 25.85750670625849068 ) ) ;
#78600=CARTESIAN_POINT ( 'NONE',  ( -2.651650429449535551, -10.15165042944956753, 18.68750000000000000 ) ) ;
#78605=CARTESIAN_POINT ( 'NONE',  ( 1.553300858899129944, -11.24999999999998934, 18.45312500000000355 ) ) ;
#78649=CARTESIAN_POINT ( 'NONE',  ( -1.553300858899125059, -3.750000000000009326, 21.57812500000000355 ) ) ;
#78694=CARTESIAN_POINT ( 'NONE',  ( 3.749999999999999556, -7.438900925035446754, 17.96688170625848713 ) ) ;
#78702=CARTESIAN_POINT ( 'NONE',  ( -3.724691934501229262, -9.114399933863657211, 19.76375670625849423 ) ) ;
#78716=CARTESIAN_POINT ( 'NONE',  ( 1.614399933863618797, -3.775308065498751198, 13.23624329374151465 ) ) ;
#78788=CARTESIAN_POINT ( 'NONE',  ( -1.553300858899125059, -3.750000000000009326, 19.07812500000000000 ) ) ;
#78798=CARTESIAN_POINT ( 'NONE',  ( -3.749999999999988454, -9.053300858899127945, 16.26562500000000000 ) ) ;
#78813=CARTESIAN_POINT ( 'NONE',  ( 0.06109907496451268821, -3.749999999999999556, 15.65811829374151287 ) ) ;
#78818=CARTESIAN_POINT ( 'NONE',  ( -2.749999999999998224, -7.500000000000015987, 22.59375000000000355 ) ) ;
#78823=CARTESIAN_POINT ( 'NONE',  ( -1.139087296525992388, -10.25000000000000711, 19.85937500000000711 ) ) ;
#78920=CARTESIAN_POINT ( 'NONE',  ( -1.901340078031369618, -5.512252781505359245, 16.75186829374151287 ) ) ;
#79031=CARTESIAN_POINT ( 'NONE',  ( -2.749999999999991562, -8.639087296526025028, 15.01562500000000178 ) ) ;
#79040=CARTESIAN_POINT ( 'NONE',  ( 1.139087296526029469, -10.24999999999999467, 14.70312500000000355 ) ) ;
#79048=CARTESIAN_POINT ( 'NONE',  ( 1.553300858899129944, -11.24999999999998934, 20.95312500000000000 ) ) ;
#79093=CARTESIAN_POINT ( 'NONE',  ( -3.749999999999988454, -9.053300858899127945, 21.26562500000000000 ) ) ;
#79099=CARTESIAN_POINT ( 'NONE',  ( 2.320192649118979489E-14, -11.25000000000000000, 17.28125000000000000 ) ) ;
#79122=MECHANICAL_DESIGN_GEOMETRIC_PRESENTATION_REPRESENTATION('',(#27318),#12973);
#79137=CARTESIAN_POINT ( 'NONE',  ( 1.492201783934554493, -3.724691934501233703, 25.23250670625849068 ) ) ;
#79146=CARTESIAN_POINT ( 'NONE',  ( 3.775308065498768517, -8.992201783934554271, 23.04500670625849068 ) ) ;
#79160=CARTESIAN_POINT ( 'NONE',  ( 3.724691934501251023, -9.114399933863618131, 13.54874329374151465 ) ) ;
#79243=CARTESIAN_POINT ( 'NONE',  ( 1.553300858899129944, -11.24999999999998934, 14.70312500000000355 ) ) ;
#79254=CARTESIAN_POINT ( 'NONE',  ( 3.750000000000009770, -9.053300858899081760, 15.79687500000000178 ) ) ;
#79270=CARTESIAN_POINT ( 'NONE',  ( 1.614399933863618797, -3.775308065498751198, 18.23624329374151642 ) ) ;
#79275=CARTESIAN_POINT ( 'NONE',  ( 1.987747218494642309, -5.598659921968629050, 13.31436829374151287 ) ) ;
#79280=CARTESIAN_POINT ( 'NONE',  ( 1.139087296526029469, -10.24999999999999289, 17.20312500000000000 ) ) ;
#79373=CARTESIAN_POINT ( 'NONE',  ( 2.775308065498755195, -6.422011778438505125, 17.14249329374151287 ) ) ;
#79403=SURFACE_STYLE_USAGE ( .BOTH. , #45605 ) ;
#79486=CARTESIAN_POINT ( 'NONE',  ( 1.139087296526029469, -10.24999999999999467, 14.70312500000000355 ) ) ;
#79495=CARTESIAN_POINT ( 'NONE',  ( -1.901340078031346525, -9.487747218494661183, 27.18563170625849068 ) ) ;
#79504=CARTESIAN_POINT ( 'NONE',  ( 3.750000000000009770, -9.053300858899081760, 23.29687500000000000 ) ) ;
#79549=CARTESIAN_POINT ( 'NONE',  ( 2.651650429449539104, -4.848349570550432475, 19.31250000000000000 ) ) ;
#79556=CARTESIAN_POINT ( 'NONE',  ( 1.553300858899129722, -11.24999999999999112, 17.20312500000000000 ) ) ;
#79588=CARTESIAN_POINT ( 'NONE',  ( 2.608446859217893099, -4.805146000318787358, 24.06063170625849423 ) ) ;
#79596=CARTESIAN_POINT ( 'NONE',  ( -3.775308065498766297, -6.007798216065450170, 24.92000670625849068 ) ) ;
#79609=CARTESIAN_POINT ( 'NONE',  ( -2.608446859217920633, -4.805146000318815780, 20.50186829374151287 ) ) ;
#79690=CARTESIAN_POINT ( 'NONE',  ( -2.651650429449565305, -4.848349570550461785, 21.50000000000000000 ) ) ;
#79700=CARTESIAN_POINT ( 'NONE',  ( -2.651650429449535551, -10.15165042944956753, 23.68750000000000000 ) ) ;
#79721=CARTESIAN_POINT ( 'NONE',  ( -2.749999999999991562, -8.639087296526025028, 26.26562500000000000 ) ) ;
#79726=CARTESIAN_POINT ( 'NONE',  ( -1.139087296525992388, -10.25000000000000711, 21.10937500000000000 ) ) ;
#79825=CARTESIAN_POINT ( 'NONE',  ( -2.724691934501246582, -6.299813628509474128, 16.67374329374151998 ) ) ;
#79925=CARTESIAN_POINT ( 'NONE',  ( 1.799775606325937360E-14, -10.25000000000000000, 16.03125000000000000 ) ) ;
#79936=CARTESIAN_POINT ( 'NONE',  ( -2.775308065498764964, -6.422011778438537988, 26.17000670625849068 ) ) ;
#79944=CARTESIAN_POINT ( 'NONE',  ( 1.553300858899087311, -3.749999999999992006, 22.98437500000000000 ) ) ;
#79992=CARTESIAN_POINT ( 'NONE',  ( 2.651650429449569302, -10.15165042944953733, 17.12500000000000000 ) ) ;
#80024=CARTESIAN_POINT ( 'NONE',  ( 2.694853999681214862, -10.10844685921789043, 26.87313170625849423 ) ) ;
#80036=CARTESIAN_POINT ( 'NONE',  ( 1.492201783934554493, -3.724691934501233703, 25.23250670625849068 ) ) ;
#80049=CARTESIAN_POINT ( 'NONE',  ( -3.724691934501248802, -5.885600066136383646, 20.42374329374152353 ) ) ;
#80134=CARTESIAN_POINT ( 'NONE',  ( -1.553300858899125059, -3.750000000000009326, 21.57812500000000355 ) ) ;
#80145=CARTESIAN_POINT ( 'NONE',  ( 1.553300858899087311, -3.749999999999992006, 22.98437500000000000 ) ) ;
#80165=CARTESIAN_POINT ( 'NONE',  ( 1.200186371490529202, -4.775308065498752974, 15.73624329374151998 ) ) ;
#80172=CARTESIAN_POINT ( 'NONE',  ( -1.409462824231155764E-14, -4.749999999999999112, 16.65625000000000000 ) ) ;
#80268=CARTESIAN_POINT ( 'NONE',  ( -1.200186371490524317, -10.22469193450124791, 13.86124329374151820 ) ) ;
#80383=CARTESIAN_POINT ( 'NONE',  ( -2.775308065498764964, -6.422011778438537988, 26.17000670625849068 ) ) ;
#80391=CARTESIAN_POINT ( 'NONE',  ( -2.749999999999991562, -8.639087296526025028, 15.01562500000000178 ) ) ;
#80399=CARTESIAN_POINT ( 'NONE',  ( 1.553300858899087311, -3.749999999999992006, 21.73437500000000000 ) ) ;
#80448=CARTESIAN_POINT ( 'NONE',  ( 3.750000000000000888, -7.499999999999978684, 16.96875000000000000 ) ) ;
#80477=CARTESIAN_POINT ( 'NONE',  ( -3.749999999999996447, -7.561099074964554134, 27.34188170625848713 ) ) ;
#80488=CARTESIAN_POINT ( 'NONE',  ( 2.608446859217893099, -4.805146000318787358, 26.56063170625849068 ) ) ;
#80504=CARTESIAN_POINT ( 'NONE',  ( 2.608446859217924629, -10.19485399968118422, 18.62686829374151642 ) ) ;
#80521=DIRECTION ( 'NONE',  ( 1.000000000000000000, 0.000000000000000000, -0.000000000000000000 ) ) ;
#80593=CARTESIAN_POINT ( 'NONE',  ( -3.749999999999997335, -7.500000000000021316, 23.84375000000000000 ) ) ;
#80601=CARTESIAN_POINT ( 'NONE',  ( 1.553300858899087311, -3.749999999999992006, 24.23437500000000355 ) ) ;
#80620=CARTESIAN_POINT ( 'NONE',  ( 2.750000000000002665, -7.561099074964516831, 17.22061829374151287 ) ) ;
#80628=CARTESIAN_POINT ( 'NONE',  ( -1.944543648262992530, -9.444543648263016067, 22.43750000000000000 ) ) ;
#80643=ORIENTED_EDGE ( 'NONE', *, *, #38124, .F. ) ;
#80726=CARTESIAN_POINT ( 'NONE',  ( 1.077988221561497539, -10.27530806549875386, 19.95499329374151642 ) ) ;
#80810=CARTESIAN_POINT ( 'NONE',  ( -1.929879867024197893E-14, -3.750000000000000000, 14.15625000000000000 ) ) ;
#80833=CARTESIAN_POINT ( 'NONE',  ( 2.750000000000001332, -7.438900925035452083, 26.71688170625849068 ) ) ;
#80841=CARTESIAN_POINT ( 'NONE',  ( -0.06109907496454585613, -4.750000000000000000, 26.40438170625848713 ) ) ;
#80850=CARTESIAN_POINT ( 'NONE',  ( -3.750000000000008438, -5.946699141100917352, 22.67187500000000355 ) ) ;
#80885=APPLICATION_CONTEXT ( 'automotive_design' ) ;
#80899=CARTESIAN_POINT ( 'NONE',  ( -1.553300858899081760, -11.25000000000000888, 14.85937500000000355 ) ) ;
#80929=CARTESIAN_POINT ( 'NONE',  ( 3.724691934501232815, -5.885600066136343678, 22.88875670625849068 ) ) ;
#80942=CARTESIAN_POINT ( 'NONE',  ( 3.749999999999999556, -7.438900925035446754, 25.46688170625849423 ) ) ;
#80950=CARTESIAN_POINT ( 'NONE',  ( -2.694853999681181556, -10.10844685921792241, 20.18936829374151287 ) ) ;
#80957=CARTESIAN_POINT ( 'NONE',  ( 1.614399933863618797, -3.775308065498751198, 20.73624329374151287 ) ) ;
#81035=CARTESIAN_POINT ( 'NONE',  ( 1.553300858899087311, -3.749999999999992006, 24.23437500000000355 ) ) ;
#81043=CARTESIAN_POINT ( 'NONE',  ( 3.750000000000009770, -9.053300858899081760, 22.04687500000000000 ) ) ;
#81056=EDGE_CURVE ( 'NONE', #61929, #73515, #86339, .T. ) ;
#81060=CARTESIAN_POINT ( 'NONE',  ( -1.987747218494638313, -9.401340078031370950, 18.93936829374151287 ) ) ;
#81069=CARTESIAN_POINT ( 'NONE',  ( -1.139087296526025250, -4.750000000000006217, 25.32812500000000355 ) ) ;
#81162=CARTESIAN_POINT ( 'NONE',  ( 1.200186371490529202, -4.775308065498752974, 19.48624329374152353 ) ) ;
#81226=DIRECTION ( 'NONE',  ( 1.000000000000000000, 0.000000000000000000, 0.000000000000000000 ) ) ;
#81267=CARTESIAN_POINT ( 'NONE',  ( 2.749999999999995115, -6.360912703473971419, 20.64062500000000000 ) ) ;
#81277=CARTESIAN_POINT ( 'NONE',  ( 1.139087296525997273, -4.749999999999992895, 20.48437500000000000 ) ) ;
#81337=CARTESIAN_POINT ( 'NONE',  ( -2.651650429449565305, -4.848349570550461785, 19.00000000000000000 ) ) ;
#81365=CARTESIAN_POINT ( 'NONE',  ( -1.901340078031346525, -9.487747218494661183, 17.18563170625848713 ) ) ;
#81380=CARTESIAN_POINT ( 'NONE',  ( -3.724691934501229262, -9.114399933863657211, 26.01375670625848713 ) ) ;
#81388=CARTESIAN_POINT ( 'NONE',  ( 3.724691934501251023, -9.114399933863618131, 17.29874329374151642 ) ) ;
#81395=CARTESIAN_POINT ( 'NONE',  ( 1.492201783934598236, -11.27530806549875031, 21.20499329374151998 ) ) ;
#81410=DIRECTION ( 'NONE',  ( 0.000000000000000000, 0.000000000000000000, 1.000000000000000000 ) ) ;
#81478=CARTESIAN_POINT ( 'NONE',  ( -1.553300858899081538, -11.25000000000000711, 19.85937500000000355 ) ) ;
#81488=CARTESIAN_POINT ( 'NONE',  ( -3.749999999999997335, -7.500000000000021316, 21.34375000000000000 ) ) ;
#81499=ORIENTED_EDGE ( 'NONE', *, *, #22476, .T. ) ;
#81502=CARTESIAN_POINT ( 'NONE',  ( 2.750000000000002665, -7.561099074964516831, 15.97061829374151287 ) ) ;
#81508=CARTESIAN_POINT ( 'NONE',  ( 2.749999999999995115, -6.360912703473971419, 23.14062499999999645 ) ) ;
#81601=CARTESIAN_POINT ( 'NONE',  ( -2.724691934501246582, -6.299813628509474128, 21.67374329374151287 ) ) ;
#81706=DIRECTION ( 'NONE',  ( -0.7071067811865510144, 0.7071067811865441310, 0.000000000000000000 ) ) ;
#81708=CARTESIAN_POINT ( 'NONE',  ( -2.749999999999991562, -8.639087296526025028, 20.01562500000000355 ) ) ;
#81718=CARTESIAN_POINT ( 'NONE',  ( 1.944543648263018731, -9.444543648262994751, 22.12500000000000000 ) ) ;
#81727=CARTESIAN_POINT ( 'NONE',  ( -2.651650429449565305, -4.848349570550461785, 25.25000000000000000 ) ) ;
#81777=CARTESIAN_POINT ( 'NONE',  ( -2.651650429449565305, -4.848349570550461785, 20.25000000000000000 ) ) ;
#81808=CARTESIAN_POINT ( 'NONE',  ( 2.750000000000001332, -7.438900925035452083, 16.71688170625848713 ) ) ;
#81821=CARTESIAN_POINT ( 'NONE',  ( 1.901340078031349856, -5.512252781505337929, 19.06063170625849068 ) ) ;
#81829=CARTESIAN_POINT ( 'NONE',  ( -0.06109907496450878162, -11.25000000000000000, 21.28311829374151287 ) ) ;
#81834=CARTESIAN_POINT ( 'NONE',  ( 3.724691934501251023, -9.114399933863618131, 24.79874329374151998 ) ) ;
#81920=CARTESIAN_POINT ( 'NONE',  ( -2.608446859217889546, -10.19485399968121264, 17.18563170625848713 ) ) ;
#81930=CARTESIAN_POINT ( 'NONE',  ( -2.694853999681210865, -4.891553140782108677, 17.49813170625848713 ) ) ;
#81947=CARTESIAN_POINT ( 'NONE',  ( -2.724691934501246582, -6.299813628509474128, 15.42374329374151642 ) ) ;
#81953=CARTESIAN_POINT ( 'NONE',  ( 1.139087296526029469, -10.24999999999999289, 22.20312500000000000 ) ) ;
#82047=CARTESIAN_POINT ( 'NONE',  ( 2.750000000000002665, -7.561099074964516831, 19.72061829374151287 ) ) ;
#82052=SURFACE_STYLE_USAGE ( .BOTH. , #54558 ) ;
#82093=B_SPLINE_CURVE_WITH_KNOTS ( 'NONE', 3,
 ( #83138, #48896, #35838, #70054, #8364, #35383, #22315, #49779, #77254, #15564, #68284, #30839, #78584, #50661, #70947, #50211, #72271, #16885, #71375, #36282, #84472, #63738, #64612, #56979, #8809, #51090, #30403, #58761, #57870, #9258, #23200, #78143, #43914, #16007, #16445, #2039, #10583, #36715, #77697, #38050, #31294, #85354 ),
 .UNSPECIFIED., .F., .F.,
 ( 4, 2, 2, 2, 2, 2, 2, 2, 2, 2, 2, 2, 2, 2, 2, 2, 2, 2, 2, 2, 4 ),
 ( 0.000000000000000000, 0.0006451441852033102092, 0.001290288370406620418, 0.001935432555609930627, 0.002580576740813240403, 0.003870865111219860388, 0.005161153481626479939, 0.005806297666829790365, 0.006451441852033101658, 0.007096586037236412951, 0.007741730222439724245, 0.008386874407643036405, 0.008709446500244692052, 0.009032018592846349433, 0.009112661615996761610, 0.009193304639147175522, 0.009233626150722380743, 0.009273947662297585964, 0.009354590685448003345, 0.009677162778049660727, 0.01032230696325297896 ),
 .UNSPECIFIED. ) ;
#82152=CARTESIAN_POINT ( 'NONE',  ( 2.750000000000001776, -7.499999999999984013, 16.96875000000000000 ) ) ;
#82161=CARTESIAN_POINT ( 'NONE',  ( 1.139087296526029469, -10.24999999999999467, 18.45312500000000355 ) ) ;
#82218=CARTESIAN_POINT ( 'NONE',  ( 3.750000000000000888, -7.499999999999978684, 19.46875000000000000 ) ) ;
#82249=CARTESIAN_POINT ( 'NONE',  ( 2.775308065498768517, -8.577988221561467341, 15.54500670625849246 ) ) ;
#82263=CARTESIAN_POINT ( 'NONE',  ( 2.724691934501235036, -6.299813628509441266, 19.13875670625849068 ) ) ;
#82270=CARTESIAN_POINT ( 'NONE',  ( 3.724691934501251023, -9.114399933863618131, 21.04874329374151642 ) ) ;
#82277=CARTESIAN_POINT ( 'NONE',  ( 3.724691934501251023, -9.114399933863618131, 22.29874329374151642 ) ) ;
#82361=CARTESIAN_POINT ( 'NONE',  ( -3.750000000000008438, -5.946699141100917352, 26.42187500000000000 ) ) ;
#82370=CARTESIAN_POINT ( 'NONE',  ( -1.614399933863656544, -3.775308065498769405, 16.32625670625849068 ) ) ;
#82385=CARTESIAN_POINT ( 'NONE',  ( -0.06109907496451398579, -10.25000000000000178, 20.03311829374151287 ) ) ;
#82392=CARTESIAN_POINT ( 'NONE',  ( 1.944543648263018731, -9.444543648262994751, 25.87500000000000355 ) ) ;
#82494=CARTESIAN_POINT ( 'NONE',  ( -1.077988221561493543, -4.724691934501247914, 18.07999329374151287 ) ) ;
#82553=CARTESIAN_POINT ( 'NONE',  ( 1.553300858899129944, -11.24999999999998934, 25.95312500000000000 ) ) ;
#82603=CARTESIAN_POINT ( 'NONE',  ( -2.749999999999998224, -7.500000000000015987, 21.34375000000000000 ) ) ;
#82615=CARTESIAN_POINT ( 'NONE',  ( 2.750000000000008438, -8.639087296525996607, 18.29687500000000000 ) ) ;
#82670=CARTESIAN_POINT ( 'NONE',  ( -1.553300858899125059, -3.750000000000009326, 19.07812500000000000 ) ) ;
#82698=CARTESIAN_POINT ( 'NONE',  ( -1.987747218494660295, -5.598659921968651254, 16.24813170625848713 ) ) ;
#82709=CARTESIAN_POINT ( 'NONE',  ( 1.200186371490561621, -10.22469193450123193, 20.70125670625849423 ) ) ;
#82716=CARTESIAN_POINT ( 'NONE',  ( 3.750000000000001776, -7.561099074964511502, 23.47061829374151642 ) ) ;
#82721=CARTESIAN_POINT ( 'NONE',  ( 3.750000000000009770, -9.053300858899081760, 14.54687500000000178 ) ) ;
#82805=CARTESIAN_POINT ( 'NONE',  ( 1.492201783934554493, -3.724691934501233703, 16.48250670625849423 ) ) ;
#82814=CARTESIAN_POINT ( 'NONE',  ( -3.724691934501229262, -9.114399933863657211, 18.51375670625849068 ) ) ;
#82829=CARTESIAN_POINT ( 'NONE',  ( 1.901340078031373171, -9.487747218494639867, 23.62686829374151287 ) ) ;
#82916=CARTESIAN_POINT ( 'NONE',  ( 3.750000000000009770, -9.053300858899081760, 14.54687500000000178 ) ) ;
#82930=CARTESIAN_POINT ( 'NONE',  ( -0.06109907496451398579, -10.25000000000000178, 25.03311829374151287 ) ) ;
#83033=CARTESIAN_POINT ( 'NONE',  ( 1.799775606325937360E-14, -10.25000000000000000, 17.28125000000000000 ) ) ;
#83052=CARTESIAN_POINT ( 'NONE',  ( 1.553300858899129944, -11.24999999999998934, 25.95312500000000000 ) ) ;
#83103=CARTESIAN_POINT ( 'NONE',  ( 1.553300858899086867, -3.749999999999992006, 17.98437500000000000 ) ) ;
#83135=CARTESIAN_POINT ( 'NONE',  ( -1.077988221561460236, -10.27530806549876452, 19.60750670625849068 ) ) ;
#83138=CARTESIAN_POINT ( 'NONE',  ( -2.651650429449565305, -4.848349570550461785, 14.00000000000000178 ) ) ;
#83146=CARTESIAN_POINT ( 'NONE',  ( 0.06109907496454976272, -10.25000000000000000, 20.77938170625848713 ) ) ;
#83153=CARTESIAN_POINT ( 'NONE',  ( -1.492201783934593573, -3.724691934501250135, 24.32999329374151642 ) ) ;
#83161=CARTESIAN_POINT ( 'NONE',  ( -0.06109907496450878162, -11.25000000000000000, 22.53311829374151642 ) ) ;
#83241=CARTESIAN_POINT ( 'NONE',  ( -1.614399933863656544, -3.775308065498769405, 15.07625670625849068 ) ) ;
#83252=CARTESIAN_POINT ( 'NONE',  ( 3.724691934501232815, -5.885600066136343678, 16.63875670625849068 ) ) ;
#83260=AXIS2_PLACEMENT_3D ( 'NONE', #63288, #84029, #77690 ) ;
#83269=CARTESIAN_POINT ( 'NONE',  ( -1.987747218494638313, -9.401340078031370950, 22.68936829374151287 ) ) ;
#83372=ADVANCED_FACE ( 'NONE', ( #42818 ), #35742, .T. ) ;
#83374=CARTESIAN_POINT ( 'NONE',  ( 1.901340078031373171, -9.487747218494639867, 24.87686829374151642 ) ) ;
#83448=AXIS2_PLACEMENT_3D ( 'NONE', #62763, #83959, #35307 ) ;
#83486=CARTESIAN_POINT ( 'NONE',  ( 1.139087296526029469, -10.24999999999999467, 25.95312500000000000 ) ) ;
#83555=CARTESIAN_POINT ( 'NONE',  ( 3.749999999999992006, -5.946699141100872943, 24.39062500000000000 ) ) ;
#83559=MECHANICAL_DESIGN_GEOMETRIC_PRESENTATION_REPRESENTATION('',(#74701),#72159);
#83592=CARTESIAN_POINT ( 'NONE',  ( 1.200186371490561621, -10.22469193450123193, 24.45125670625849423 ) ) ;
#83603=CARTESIAN_POINT ( 'NONE',  ( 2.750000000000001332, -7.438900925035452083, 16.71688170625848713 ) ) ;
#83610=CARTESIAN_POINT ( 'NONE',  ( -0.06109907496450878162, -11.25000000000000000, 22.53311829374151642 ) ) ;
#83615=CARTESIAN_POINT ( 'NONE',  ( 2.694853999681185108, -4.891553140782077591, 22.06436829374151287 ) ) ;
#83696=CARTESIAN_POINT ( 'NONE',  ( 3.750000000000000888, -7.499999999999978684, 25.71875000000000000 ) ) ;
#83705=CARTESIAN_POINT ( 'NONE',  ( 2.608446859217893099, -4.805146000318787358, 16.56063170625848713 ) ) ;
#83719=CARTESIAN_POINT ( 'NONE',  ( 1.200186371490529202, -4.775308065498752974, 20.73624329374151287 ) ) ;
#83825=CARTESIAN_POINT ( 'NONE',  ( 0.06109907496451789238, -4.749999999999998224, 24.40811829374151642 ) ) ;
#83833=CARTESIAN_POINT ( 'NONE',  ( 1.139087296525997051, -4.749999999999992895, 14.23437500000000178 ) ) ;
#83932=CARTESIAN_POINT ( 'NONE',  ( 1.799775606325937360E-14, -10.25000000000000000, 22.28125000000000355 ) ) ;
#83959=DIRECTION ( 'NONE',  ( 0.000000000000000000, 0.000000000000000000, 1.000000000000000000 ) ) ;
#83997=CARTESIAN_POINT ( 'NONE',  ( 2.651650429449569302, -10.15165042944953733, 24.62500000000000000 ) ) ;
#84029=DIRECTION ( 'NONE',  ( -0.7057856980126718804, -0.7057856980126787638, -0.06109907496453170772 ) ) ;
#84033=CARTESIAN_POINT ( 'NONE',  ( -0.06109907496454585613, -4.750000000000000000, 21.40438170625849068 ) ) ;
#84044=CARTESIAN_POINT ( 'NONE',  ( -0.06109907496454585613, -4.750000000000000000, 23.90438170625849068 ) ) ;
#84052=CARTESIAN_POINT ( 'NONE',  ( -1.553300858899081538, -11.25000000000000711, 18.60937500000000355 ) ) ;
#84058=CARTESIAN_POINT ( 'NONE',  ( 3.750000000000000888, -7.499999999999978684, 15.71875000000000000 ) ) ;
#84141=CARTESIAN_POINT ( 'NONE',  ( 1.492201783934554493, -3.724691934501233703, 20.23250670625849423 ) ) ;
#84150=CARTESIAN_POINT ( 'NONE',  ( -1.492201783934549164, -11.27530806549876807, 20.85750670625849068 ) ) ;
#84163=CARTESIAN_POINT ( 'NONE',  ( 1.987747218494642309, -5.598659921968629050, 23.31436829374150932 ) ) ;
#84244=CARTESIAN_POINT ( 'NONE',  ( -3.750000000000008438, -5.946699141100917352, 15.17187500000000000 ) ) ;
#84268=CARTESIAN_POINT ( 'NONE',  ( 0.06109907496451789238, -4.749999999999998224, 23.15811829374151642 ) ) ;
#84273=CARTESIAN_POINT ( 'NONE',  ( -2.749999999999998224, -7.500000000000015987, 20.09375000000000000 ) ) ;
#84279=CARTESIAN_POINT ( 'NONE',  ( 2.750000000000008438, -8.639087296525996607, 15.79687500000000178 ) ) ;
#84370=CARTESIAN_POINT ( 'NONE',  ( 1.139087296526029469, -10.24999999999999467, 23.45312500000000000 ) ) ;
#84440=CARTESIAN_POINT ( 'NONE',  ( 1.553300858899129722, -11.24999999999999112, 25.95312500000000000 ) ) ;
#84470=CARTESIAN_POINT ( 'NONE',  ( 2.724691934501235036, -6.299813628509441266, 21.63875670625848713 ) ) ;
#84472=CARTESIAN_POINT ( 'NONE',  ( 3.375057480660595299, -6.401003086717466317, 14.00000000000007994 ) ) ;
#84481=CARTESIAN_POINT ( 'NONE',  ( 2.724691934501235036, -6.299813628509441266, 25.38875670625849423 ) ) ;
#84489=CARTESIAN_POINT ( 'NONE',  ( -3.749999999999997335, -7.500000000000021316, 15.09375000000000000 ) ) ;
#84494=CARTESIAN_POINT ( 'NONE',  ( -3.750000000000008438, -5.946699141100917352, 17.67187500000000355 ) ) ;
#84535=CARTESIAN_POINT ( 'NONE',  ( 2.651650429449569302, -10.15165042944953733, 20.87500000000000000 ) ) ;
#84580=CARTESIAN_POINT ( 'NONE',  ( 0.06109907496455496689, -11.24999999999999822, 19.52938170625848713 ) ) ;
#84589=CARTESIAN_POINT ( 'NONE',  ( 3.724691934501232815, -5.885600066136343678, 19.13875670625849068 ) ) ;
#84604=CARTESIAN_POINT ( 'NONE',  ( -1.901340078031369618, -5.512252781505359245, 25.50186829374151287 ) ) ;
#84686=CARTESIAN_POINT ( 'NONE',  ( -3.749999999999988454, -9.053300858899127945, 18.76562500000000000 ) ) ;
#84695=CARTESIAN_POINT ( 'NONE',  ( 2.651650429449539104, -4.848349570550432475, 19.31250000000000000 ) ) ;
#84712=CARTESIAN_POINT ( 'NONE',  ( -1.077988221561493543, -4.724691934501247914, 24.32999329374151642 ) ) ;
#84718=CARTESIAN_POINT ( 'NONE',  ( 1.139087296526029469, -10.24999999999999467, 23.45312500000000000 ) ) ;
#84722=CARTESIAN_POINT ( 'NONE',  ( -2.749999999999991562, -8.639087296526026805, 16.26562500000000000 ) ) ;
#84819=CARTESIAN_POINT ( 'NONE',  ( 2.750000000000008438, -8.639087296525996607, 25.79687500000000355 ) ) ;
#84914=CARTESIAN_POINT ( 'NONE',  ( 1.987747218494664292, -9.401340078031346081, 23.12313170625848713 ) ) ;
#84926=CARTESIAN_POINT ( 'NONE',  ( -1.200186371490556958, -4.775308065498765409, 22.57625670625848713 ) ) ;
#84935=CARTESIAN_POINT ( 'NONE',  ( 2.651650429449569302, -10.15165042944953733, 17.12500000000000000 ) ) ;
#84939=CARTESIAN_POINT ( 'NONE',  ( 3.750000000000009770, -9.053300858899081760, 18.29687500000000000 ) ) ;
#84973=CARTESIAN_POINT ( 'NONE',  ( -3.749999999999997335, -7.500000000000021316, 20.09375000000000000 ) ) ;
#85015=CARTESIAN_POINT ( 'NONE',  ( 3.775308065498768517, -8.992201783934554271, 18.04500670625848713 ) ) ;
#85023=CARTESIAN_POINT ( 'NONE',  ( 1.492201783934554493, -3.724691934501233703, 21.48250670625849068 ) ) ;
#85039=CARTESIAN_POINT ( 'NONE',  ( -3.775308065498748977, -8.992201783934593351, 14.01749329374151642 ) ) ;
#85116=CARTESIAN_POINT ( 'NONE',  ( 1.553300858899087311, -3.749999999999992006, 17.98437500000000000 ) ) ;
#85127=CARTESIAN_POINT ( 'NONE',  ( 2.320192649118979489E-14, -11.25000000000000000, 19.78125000000000000 ) ) ;
#85142=CARTESIAN_POINT ( 'NONE',  ( 2.694853999681185108, -4.891553140782077591, 18.31436829374150932 ) ) ;
#85146=CARTESIAN_POINT ( 'NONE',  ( 1.944543648263018731, -9.444543648262994751, 25.87500000000000355 ) ) ;
#85150=CARTESIAN_POINT ( 'NONE',  ( 1.139087296526029469, -10.24999999999999289, 19.70312500000000355 ) ) ;
#85249=CARTESIAN_POINT ( 'NONE',  ( 1.944543648262996083, -5.555456351736983045, 24.31250000000000000 ) ) ;
#85351=CARTESIAN_POINT ( 'NONE',  ( -1.901340078031346525, -9.487747218494661183, 23.43563170625848713 ) ) ;
#85354=CARTESIAN_POINT ( 'NONE',  ( 2.952004793765244717, -6.965521097154411478, 14.00000000000000178 ) ) ;
#85362=CARTESIAN_POINT ( 'NONE',  ( -2.749999999999997780, -7.561099074964547917, 24.84188170625848713 ) ) ;
#85370=CARTESIAN_POINT ( 'NONE',  ( 3.750000000000000888, -7.499999999999978684, 18.21875000000000000 ) ) ;
#85375=CARTESIAN_POINT ( 'NONE',  ( 2.651650429449569302, -10.15165042944953733, 15.87500000000000000 ) ) ;
#85413=CARTESIAN_POINT ( 'NONE',  ( -3.749999999999997335, -7.500000000000021316, 23.84375000000000000 ) ) ;
#85451=CARTESIAN_POINT ( 'NONE',  ( 3.724691934501232815, -5.885600066136343678, 21.63875670625848713 ) ) ;
#85459=CARTESIAN_POINT ( 'NONE',  ( -0.06109907496455085213, -3.750000000000000888, 20.15438170625849068 ) ) ;
#85473=CARTESIAN_POINT ( 'NONE',  ( -0.06109907496451398579, -10.25000000000000178, 25.03311829374151287 ) ) ;
#85555=CARTESIAN_POINT ( 'NONE',  ( 2.651650429449569302, -10.15165042944953733, 18.37500000000000355 ) ) ;
#85565=CARTESIAN_POINT ( 'NONE',  ( -2.651650429449535551, -10.15165042944956753, 16.18750000000000000 ) ) ;
#85580=CARTESIAN_POINT ( 'NONE',  ( 1.614399933863618797, -3.775308065498751198, 16.98624329374151287 ) ) ;
#85585=CARTESIAN_POINT ( 'NONE',  ( 0.06109907496451789238, -4.749999999999998224, 13.15811829374151642 ) ) ;
#85589=CARTESIAN_POINT ( 'NONE',  ( 2.749999999999995115, -6.360912703473971419, 16.89062500000000000 ) ) ;
#85688=CARTESIAN_POINT ( 'NONE',  ( 1.987747218494642309, -5.598659921968629050, 13.31436829374151287 ) ) ;
#85716=FILL_AREA_STYLE_COLOUR ( '', #53213 ) ;
#85800=CARTESIAN_POINT ( 'NONE',  ( 1.200186371490561621, -10.22469193450123193, 25.70125670625848713 ) ) ;
#85809=CARTESIAN_POINT ( 'NONE',  ( -1.901340078031346525, -9.487747218494661183, 23.43563170625848713 ) ) ;
#85818=CARTESIAN_POINT ( 'NONE',  ( -3.749999999999988454, -9.053300858899127945, 15.01562500000000178 ) ) ;
#85856=CARTESIAN_POINT ( 'NONE',  ( -3.750000000000008438, -5.946699141100917352, 23.92187500000000355 ) ) ;
#85863=CARTESIAN_POINT ( 'NONE',  ( -3.749999999999988454, -9.053300858899127945, 16.26562500000000000 ) ) ;
#85897=CARTESIAN_POINT ( 'NONE',  ( 0.06109907496455496689, -11.24999999999999822, 20.77938170625848713 ) ) ;
#85905=CARTESIAN_POINT ( 'NONE',  ( -2.694853999681210865, -4.891553140782108677, 21.24813170625848713 ) ) ;
#85921=CARTESIAN_POINT ( 'NONE',  ( 1.200186371490529202, -4.775308065498752974, 24.48624329374151642 ) ) ;
#86000=CARTESIAN_POINT ( 'NONE',  ( 3.750000000000009770, -9.053300858899081760, 17.04687500000000000 ) ) ;
#86010=CARTESIAN_POINT ( 'NONE',  ( 3.750000000000000888, -7.499999999999978684, 18.21875000000000000 ) ) ;
#86027=CARTESIAN_POINT ( 'NONE',  ( 3.750000000000001776, -7.561099074964511502, 17.22061829374151287 ) ) ;
#86032=CARTESIAN_POINT ( 'NONE',  ( -2.750000000000007105, -6.360912703474006946, 26.42187500000000000 ) ) ;
#86039=CARTESIAN_POINT ( 'NONE',  ( -2.749999999999998224, -7.500000000000015987, 17.59375000000000000 ) ) ;
#86137=CARTESIAN_POINT ( 'NONE',  ( 2.775308065498755195, -6.422011778438505125, 15.89249329374151820 ) ) ;
#86230=ORIENTED_EDGE ( 'NONE', *, *, #23428, .T. ) ;
#86255=CARTESIAN_POINT ( 'NONE',  ( 1.139087296525997273, -4.749999999999992895, 14.23437500000000355 ) ) ;
#86265=CARTESIAN_POINT ( 'NONE',  ( 2.749999999999995115, -6.360912703473971419, 16.89062500000000000 ) ) ;
#86275=CARTESIAN_POINT ( 'NONE',  ( -1.553300858899081538, -11.25000000000000711, 21.10937500000000711 ) ) ;
#86318=CARTESIAN_POINT ( 'NONE',  ( 1.553300858899087311, -3.749999999999992006, 19.23437500000000355 ) ) ;
#86326=CARTESIAN_POINT ( 'NONE',  ( -1.929879867024197893E-14, -3.750000000000000000, 15.40625000000000000 ) ) ;
#86339=CIRCLE ( 'NONE', #64695, 3.000000000000000000 ) ;
#86361=CARTESIAN_POINT ( 'NONE',  ( 3.775308065498768517, -8.992201783934554271, 24.29500670625849423 ) ) ;
#86370=CARTESIAN_POINT ( 'NONE',  ( -3.724691934501229262, -9.114399933863657211, 24.76375670625848713 ) ) ;
#86385=CARTESIAN_POINT ( 'NONE',  ( -2.694853999681181556, -10.10844685921792241, 13.93936829374151465 ) ) ;
#86465=CARTESIAN_POINT ( 'NONE',  ( 3.750000000000000888, -7.499999999999978684, 20.71875000000000000 ) ) ;
#86475=CARTESIAN_POINT ( 'NONE',  ( 2.651650429449569302, -10.15165042944953733, 23.37500000000000000 ) ) ;
#86492=CARTESIAN_POINT ( 'NONE',  ( -1.944543648263014957, -5.555456351737005249, 22.75000000000000000 ) ) ;
#86497=CARTESIAN_POINT ( 'NONE',  ( 1.944543648263018731, -9.444543648262994751, 20.87500000000000000 ) ) ;
#86590=CARTESIAN_POINT ( 'NONE',  ( 2.750000000000002665, -7.561099074964516831, 17.22061829374151287 ) ) ;
#86707=CARTESIAN_POINT ( 'NONE',  ( 0.06109907496454976272, -10.25000000000000000, 27.02938170625848358 ) ) ;
#86717=CARTESIAN_POINT ( 'NONE',  ( 1.139087296525997273, -4.749999999999992895, 16.73437500000000000 ) ) ;
#86727=CARTESIAN_POINT ( 'NONE',  ( -2.651650429449535551, -10.15165042944956753, 22.43750000000000000 ) ) ;
#86761=ADVANCED_FACE ( 'NONE', ( #21864 ), #34927, .T. ) ;
#86768=CARTESIAN_POINT ( 'NONE',  ( -2.651650429449565305, -4.848349570550461785, 25.25000000000000000 ) ) ;
#86775=CARTESIAN_POINT ( 'NONE',  ( 2.651650429449569302, -10.15165042944953733, 14.62500000000000000 ) ) ;
#86808=CARTESIAN_POINT ( 'NONE',  ( -0.06109907496455085213, -3.750000000000000888, 26.40438170625848713 ) ) ;
#86820=CARTESIAN_POINT ( 'NONE',  ( 1.492201783934554493, -3.724691934501233703, 23.98250670625849068 ) ) ;
#86836=CARTESIAN_POINT ( 'NONE',  ( 3.724691934501251023, -9.114399933863618131, 17.29874329374151642 ) ) ;
#86854=PLANE ( 'NONE',  #48422 ) ;
#86918=CARTESIAN_POINT ( 'NONE',  ( -3.749999999999988454, -9.053300858899127945, 20.01562500000000355 ) ) ;
#86930=CARTESIAN_POINT ( 'NONE',  ( 3.750000000000000888, -7.499999999999978684, 21.96875000000000355 ) ) ;
#86947=CARTESIAN_POINT ( 'NONE',  ( -2.749999999999999112, -7.438900925035484057, 15.34561829374151465 ) ) ;
#86952=CARTESIAN_POINT ( 'NONE',  ( -1.139087296526025250, -4.750000000000006217, 20.32812500000000711 ) ) ;
#87042=CARTESIAN_POINT ( 'NONE',  ( -2.724691934501246582, -6.299813628509474128, 17.92374329374151287 ) ) ;
#87147=CARTESIAN_POINT ( 'NONE',  ( 1.987747218494664292, -9.401340078031346081, 25.62313170625849068 ) ) ;
#87156=CARTESIAN_POINT ( 'NONE',  ( 1.139087296525997273, -4.749999999999992895, 14.23437500000000355 ) ) ;
#87165=CARTESIAN_POINT ( 'NONE',  ( 2.320192649118979489E-14, -11.25000000000000000, 19.78125000000000000 ) ) ;
#87215=CARTESIAN_POINT ( 'NONE',  ( 1.553300858899086867, -3.749999999999992006, 15.48437499999999822 ) ) ;
#87246=CARTESIAN_POINT ( 'NONE',  ( -1.492201783934549164, -11.27530806549876807, 23.35750670625849423 ) ) ;
#87256=CARTESIAN_POINT ( 'NONE',  ( -2.749999999999997780, -7.561099074964547917, 16.09188170625848713 ) ) ;
#87270=CARTESIAN_POINT ( 'NONE',  ( 3.775308065498752086, -6.007798216065404873, 18.39249329374151642 ) ) ;
#87354=CARTESIAN_POINT ( 'NONE',  ( 3.750000000000009770, -9.053300858899081760, 22.04687500000000000 ) ) ;
#87363=CARTESIAN_POINT ( 'NONE',  ( 3.750000000000009770, -9.053300858899081760, 20.79687500000000000 ) ) ;
#87378=CARTESIAN_POINT ( 'NONE',  ( 2.775308065498755195, -6.422011778438505125, 17.14249329374151287 ) ) ;
#87385=CARTESIAN_POINT ( 'NONE',  ( -1.944543648263014957, -5.555456351737005249, 24.00000000000000000 ) ) ;
#87483=CARTESIAN_POINT ( 'NONE',  ( 1.077988221561497539, -10.27530806549875386, 13.70499329374151287 ) ) ;
#87511=( NAMED_UNIT ( * ) SI_UNIT ( $, .STERADIAN. ) SOLID_ANGLE_UNIT ( ) );
#87572=CARTESIAN_POINT ( 'NONE',  ( -2.121320343559653487, -5.378679656440369605, 14.00000000000000178 ) ) ;
#87592=CARTESIAN_POINT ( 'NONE',  ( 1.077988221561464899, -4.724691934501233703, 26.48250670625848713 ) ) ;
#87601=CARTESIAN_POINT ( 'NONE',  ( -2.749999999999997780, -7.561099074964547917, 27.34188170625848713 ) ) ;
#87608=CARTESIAN_POINT ( 'NONE',  ( -3.749999999999997335, -7.500000000000021316, 22.59375000000000355 ) ) ;
#87650=CARTESIAN_POINT ( 'NONE',  ( -3.750000000000008438, -5.946699141100917352, 26.42187500000000000 ) ) ;
#87687=CARTESIAN_POINT ( 'NONE',  ( -3.775308065498766297, -6.007798216065450170, 24.92000670625849068 ) ) ;
#87701=CARTESIAN_POINT ( 'NONE',  ( -1.492201783934549164, -11.27530806549876807, 25.85750670625849068 ) ) ;
#87712=CARTESIAN_POINT ( 'NONE',  ( 1.492201783934598236, -11.27530806549875031, 18.70499329374151287 ) ) ;
#87720=CARTESIAN_POINT ( 'NONE',  ( -3.775308065498748977, -8.992201783934593351, 16.51749329374151642 ) ) ;
#87808=CARTESIAN_POINT ( 'NONE',  ( -1.553300858899125059, -3.750000000000009326, 24.07812500000000355 ) ) ;
#87817=CARTESIAN_POINT ( 'NONE',  ( -3.749999999999988454, -9.053300858899127945, 21.26562500000000000 ) ) ;
#87834=CARTESIAN_POINT ( 'NONE',  ( -0.06109907496451398579, -10.25000000000000178, 18.78311829374151287 ) ) ;
#87843=CARTESIAN_POINT ( 'NONE',  ( 1.139087296525997051, -4.749999999999992895, 21.73437500000000000 ) ) ;
#87944=CARTESIAN_POINT ( 'NONE',  ( -2.775308065498752086, -8.577988221561495763, 21.51749329374151998 ) ) ;
#88050=CARTESIAN_POINT ( 'NONE',  ( -1.409462824231155764E-14, -4.749999999999999112, 16.65625000000000000 ) ) ;
#88060=CARTESIAN_POINT ( 'NONE',  ( 2.749999999999995115, -6.360912703473971419, 21.89062500000000355 ) ) ;
#88067=CARTESIAN_POINT ( 'NONE',  ( -1.929879867024197893E-14, -3.750000000000000000, 20.40625000000000000 ) ) ;
#88115=CARTESIAN_POINT ( 'NONE',  ( 2.651650429449539104, -4.848349570550432475, 21.81250000000000000 ) ) ;
#88141=CARTESIAN_POINT ( 'NONE',  ( 2.724691934501235036, -6.299813628509441266, 19.13875670625849068 ) ) ;
#88155=CARTESIAN_POINT ( 'NONE',  ( 2.694853999681214862, -10.10844685921789043, 24.37313170625848713 ) ) ;
#88162=CARTESIAN_POINT ( 'NONE',  ( 3.750000000000001776, -7.561099074964511502, 18.47061829374151287 ) ) ;
#88169=CARTESIAN_POINT ( 'NONE',  ( 2.694853999681185108, -4.891553140782077591, 20.81436829374151287 ) ) ;
#88251=CARTESIAN_POINT ( 'NONE',  ( -3.750000000000008438, -5.946699141100917352, 22.67187500000000355 ) ) ;
#88261=CARTESIAN_POINT ( 'NONE',  ( 2.651650429449539104, -4.848349570550432475, 24.31250000000000000 ) ) ;
#88276=CARTESIAN_POINT ( 'NONE',  ( 0.06109907496451789238, -4.749999999999998224, 15.65811829374151287 ) ) ;
#88285=CARTESIAN_POINT ( 'NONE',  ( 2.750000000000008438, -8.639087296525996607, 23.29687500000000000 ) ) ;
#88368=ORIENTED_EDGE ( 'NONE', *, *, #23428, .F. ) ;
#88376=CARTESIAN_POINT ( 'NONE',  ( 1.077988221561497539, -10.27530806549875386, 21.20499329374151998 ) ) ;
#88482=CARTESIAN_POINT ( 'NONE',  ( -1.409462824231155764E-14, -4.749999999999999112, 19.15625000000000000 ) ) ;
#88491=CARTESIAN_POINT ( 'NONE',  ( 2.750000000000001776, -7.499999999999984013, 20.71875000000000000 ) ) ;
#88499=CARTESIAN_POINT ( 'NONE',  ( -3.749999999999988454, -9.053300858899127945, 26.26562500000000000 ) ) ;
#88549=CARTESIAN_POINT ( 'NONE',  ( 2.651650429449539104, -4.848349570550432475, 19.31250000000000000 ) ) ;
#88584=CARTESIAN_POINT ( 'NONE',  ( -1.901340078031346525, -9.487747218494661183, 15.93563170625849068 ) ) ;
#88598=CARTESIAN_POINT ( 'NONE',  ( -0.06109907496454585613, -4.750000000000000000, 20.15438170625849068 ) ) ;
#88605=CARTESIAN_POINT ( 'NONE',  ( -1.614399933863613468, -11.22469193450124969, 23.86124329374151998 ) ) ;
#88610=CARTESIAN_POINT ( 'NONE',  ( -2.694853999681181556, -10.10844685921792241, 16.43936829374151287 ) ) ;
#88691=CARTESIAN_POINT ( 'NONE',  ( 2.694853999681214862, -10.10844685921789043, 16.87313170625849068 ) ) ;
#88699=CARTESIAN_POINT ( 'NONE',  ( -3.750000000000008438, -5.946699141100917352, 26.42187500000000000 ) ) ;
#88714=CARTESIAN_POINT ( 'NONE',  ( -1.901340078031369618, -5.512252781505359245, 18.00186829374151287 ) ) ;
#88721=CARTESIAN_POINT ( 'NONE',  ( -1.944543648263014957, -5.555456351737005249, 25.25000000000000000 ) ) ;
#88817=CARTESIAN_POINT ( 'NONE',  ( -1.987747218494638313, -9.401340078031370950, 22.68936829374151287 ) ) ;
#88904=CARTESIAN_POINT ( 'NONE',  ( -2.102533092329708531, -5.360057338231124291, 13.56786352175840626 ) ) ;
#88925=CARTESIAN_POINT ( 'NONE',  ( 1.944543648263018731, -9.444543648262994751, 17.12500000000000000 ) ) ;
#88935=CARTESIAN_POINT ( 'NONE',  ( -1.409462824231155764E-14, -4.749999999999999112, 19.15625000000000000 ) ) ;
#88990=CARTESIAN_POINT ( 'NONE',  ( 1.553300858899129722, -11.24999999999999112, 20.95312500000000000 ) ) ;
#89021=CARTESIAN_POINT ( 'NONE',  ( 1.077988221561464899, -4.724691934501233703, 17.73250670625848713 ) ) ;
#89033=CARTESIAN_POINT ( 'NONE',  ( 1.077988221561464899, -4.724691934501233703, 17.73250670625848713 ) ) ;
#89041=CARTESIAN_POINT ( 'NONE',  ( 0.06109907496451268821, -3.749999999999999556, 21.90811829374151642 ) ) ;
#89046=CARTESIAN_POINT ( 'NONE',  ( -2.651650429449565305, -4.848349570550461785, 14.00000000000000000 ) ) ;
#89131=CARTESIAN_POINT ( 'NONE',  ( -2.651650429449565305, -4.848349570550461785, 25.25000000000000000 ) ) ;
#89139=CARTESIAN_POINT ( 'NONE',  ( 2.320192649118979489E-14, -11.25000000000000000, 26.03125000000000000 ) ) ;
#89155=CARTESIAN_POINT ( 'NONE',  ( 2.775308065498755195, -6.422011778438505125, 20.89249329374151642 ) ) ;
#89161=CARTESIAN_POINT ( 'NONE',  ( -1.944543648262992530, -9.444543648263016067, 24.93750000000000000 ) ) ;
ENDSEC;
END-ISO-10303-21;
